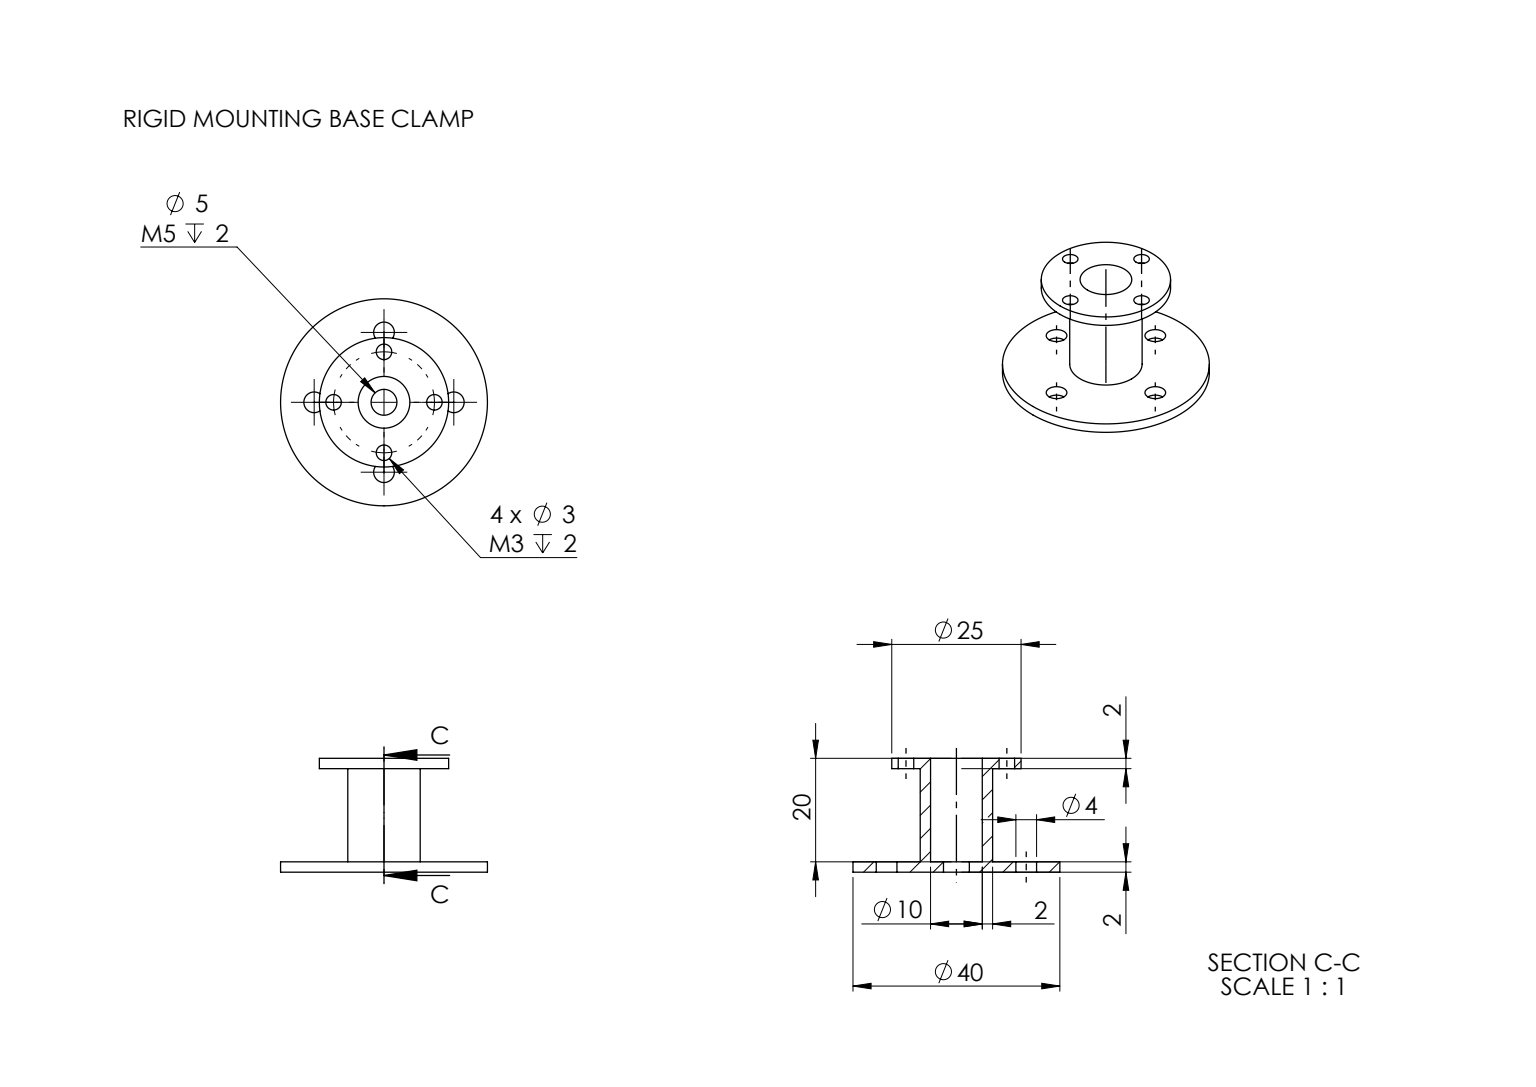
ISO-10303-21;
HEADER;
FILE_DESCRIPTION (('STEP AP214'),
    '1' );
FILE_NAME ('Rigid Mounting Base Clamp.step',
    '2026-10-04T10:31:01',
    ( '' ),
    ( '' ),
    'SwSTEP 2.0',
    'SolidWorks 2026',
    '' );
FILE_SCHEMA (( 'AUTOMOTIVE_DESIGN' ));
ENDSEC;

DATA;
#14=DIRECTION ( 'NONE',  ( 0.000000000000000000, -0.000000000000000000, 1.000000000000000000 ) ) ;
#15=DIRECTION ( 'NONE',  ( 0.000000000000000000, 1.000000000000000000, 0.000000000000000000 ) ) ;
#29=CARTESIAN_POINT ( 'NONE',  ( 8.572527594031473190E-16, 19.99999999999999645, 7.000000000000000000 ) ) ;
#45=CARTESIAN_POINT ( 'NONE',  ( 0.000000000000000000, 22.00000000000000000, -5.000000000000000000 ) ) ;
#61=ORIENTED_EDGE ( 'NONE', *, *, #6502, .F. ) ;
#68=EDGE_CURVE ( 'NONE', #7891, #15426, #13595, .T. ) ;
#80=CYLINDRICAL_SURFACE ( 'NONE', #3453, 2.000000000000000000 ) ;
#135=CARTESIAN_POINT ( 'NONE',  ( 0.000000000000000000, 2.000000000000000000, -5.000000000000000000 ) ) ;
#152=CARTESIAN_POINT ( 'NONE',  ( -13.50000000000000000, -0.001000000000000132727, -1.999999999999997113 ) ) ;
#161=ORIENTED_EDGE ( 'NONE', *, *, #15144, .T. ) ;
#168=FACE_BOUND ( 'NONE', #3506, .T. ) ;
#169=DIRECTION ( 'NONE',  ( 0.000000000000000000, 0.000000000000000000, 1.000000000000000000 ) ) ;
#211=AXIS2_PLACEMENT_3D ( 'NONE', #13271, #4928, #12230 ) ;
#214=FACE_OUTER_BOUND ( 'NONE', #10362, .T. ) ;
#234=CARTESIAN_POINT ( 'NONE',  ( 9.750000000000003553, 19.99999999999999645, 1.020968533498575335E-13 ) ) ;
#237=CYLINDRICAL_SURFACE ( 'NONE', #3717, 2.500000000000000000 ) ;
#238=CARTESIAN_POINT ( 'NONE',  ( 13.50000000000000000, 2.000000000000000000, -2.000000000000000444 ) ) ;
#241=ORIENTED_EDGE ( 'NONE', *, *, #4453, .T. ) ;
#244=AXIS2_PLACEMENT_3D ( 'NONE', #12080, #1179, #6133 ) ;
#246=CIRCLE ( 'NONE', #4794, 1.499999999999999556 ) ;
#275=EDGE_CURVE ( 'NONE', #9042, #302, #14114, .T. ) ;
#302=VERTEX_POINT ( 'NONE', #12936 ) ;
#313=DIRECTION ( 'NONE',  ( 0.000000000000000000, 0.000000000000000000, -1.000000000000000000 ) ) ;
#343=AXIS2_PLACEMENT_3D ( 'NONE', #14019, #15537, #15300 ) ;
#391=AXIS2_PLACEMENT_3D ( 'NONE', #8568, #1379, #7592 ) ;
#450=LINE ( 'NONE', #2848, #4783 ) ;
#460=EDGE_CURVE ( 'NONE', #3041, #9290, #14361, .T. ) ;
#491=AXIS2_PLACEMENT_3D ( 'NONE', #7668, #1615, #14760 ) ;
#538=( LENGTH_UNIT ( ) NAMED_UNIT ( * ) SI_UNIT ( .MILLI., .METRE. ) );
#545=DIRECTION ( 'NONE',  ( -0.000000000000000000, 1.000000000000000000, -0.000000000000000000 ) ) ;
#570=ORIENTED_EDGE ( 'NONE', *, *, #4975, .F. ) ;
#579=CIRCLE ( 'NONE', #3127, 2.500000000000000000 ) ;
#603=DIRECTION ( 'NONE',  ( 0.000000000000000000, 1.000000000000000000, 0.000000000000000000 ) ) ;
#612=VECTOR ( 'NONE', #7149, 1000.000000000000000 ) ;
#635=EDGE_CURVE ( 'NONE', #13364, #1681, #12596, .T. ) ;
#644=DIRECTION ( 'NONE',  ( 0.000000000000000000, 0.000000000000000000, 1.000000000000000000 ) ) ;
#645=VERTEX_POINT ( 'NONE', #6427 ) ;
#662=DIRECTION ( 'NONE',  ( -0.000000000000000000, 1.000000000000000000, -0.000000000000000000 ) ) ;
#688=AXIS2_PLACEMENT_3D ( 'NONE', #3084, #7934, #12777 ) ;
#703=VERTEX_POINT ( 'NONE', #13060 ) ;
#711=AXIS2_PLACEMENT_3D ( 'NONE', #4234, #3121, #10361 ) ;
#722=ORIENTED_EDGE ( 'NONE', *, *, #3306, .T. ) ;
#729=ADVANCED_FACE ( 'NONE', ( #11618 ), #5821, .F. ) ;
#732=CARTESIAN_POINT ( 'NONE',  ( -13.50000000000000000, 0.000000000000000000, 2.479909768273400161E-15 ) ) ;
#750=FACE_OUTER_BOUND ( 'NONE', #5902, .T. ) ;
#756=DIRECTION ( 'NONE',  ( 0.000000000000000000, 1.000000000000000000, 0.000000000000000000 ) ) ;
#769=ORIENTED_EDGE ( 'NONE', *, *, #11126, .T. ) ;
#798=DIRECTION ( 'NONE',  ( -0.000000000000000000, 1.000000000000000000, -0.000000000000000000 ) ) ;
#799=DIRECTION ( 'NONE',  ( 0.000000000000000000, 0.000000000000000000, 1.000000000000000000 ) ) ;
#807=( NAMED_UNIT ( * ) PLANE_ANGLE_UNIT ( ) SI_UNIT ( $, .RADIAN. ) );
#824=ORIENTED_EDGE ( 'NONE', *, *, #635, .T. ) ;
#827=DIRECTION ( 'NONE',  ( 0.000000000000000000, -0.000000000000000000, 1.000000000000000000 ) ) ;
#831=CARTESIAN_POINT ( 'NONE',  ( 0.000000000000000000, 19.99999999999999645, 12.50000000000000355 ) ) ;
#838=ADVANCED_FACE ( 'NONE', ( #7404 ), #80, .F. ) ;
#849=AXIS2_PLACEMENT_3D ( 'NONE', #732, #12900, #2001 ) ;
#852=( NAMED_UNIT ( * ) SI_UNIT ( $, .STERADIAN. ) SOLID_ANGLE_UNIT ( ) );
#866=CARTESIAN_POINT ( 'NONE',  ( 0.000000000000000000, 2.000000000000000000, -2.500000000000000000 ) ) ;
#894=EDGE_LOOP ( 'NONE', ( #6085, #14105 ) ) ;
#901=FACE_BOUND ( 'NONE', #10404, .T. ) ;
#907=CARTESIAN_POINT ( 'NONE',  ( 0.000000000000000000, 0.000000000000000000, 0.000000000000000000 ) ) ;
#919=DIRECTION ( 'NONE',  ( 0.000000000000000000, 1.000000000000000000, 0.000000000000000000 ) ) ;
#929=CARTESIAN_POINT ( 'NONE',  ( -9.750000000000003553, 22.00000000000000000, -1.500000000000033751 ) ) ;
#958=ADVANCED_FACE ( 'NONE', ( #14875 ), #237, .F. ) ;
#959=ORIENTED_EDGE ( 'NONE', *, *, #1371, .T. ) ;
#960=ORIENTED_EDGE ( 'NONE', *, *, #11186, .T. ) ;
#966=CARTESIAN_POINT ( 'NONE',  ( 9.750000000000003553, 22.00000000000000000, 1.500000000000101696 ) ) ;
#977=CIRCLE ( 'NONE', #711, 2.000000000000000000 ) ;
#978=ORIENTED_EDGE ( 'NONE', *, *, #14189, .T. ) ;
#984=DIRECTION ( 'NONE',  ( -0.000000000000000000, 1.000000000000000000, -0.000000000000000000 ) ) ;
#1005=CYLINDRICAL_SURFACE ( 'NONE', #3266, 20.00000000000000000 ) ;
#1031=CARTESIAN_POINT ( 'NONE',  ( 9.750000000000003553, 22.00000000000000000, 1.500000000000101696 ) ) ;
#1038=ORIENTED_EDGE ( 'NONE', *, *, #14388, .F. ) ;
#1040=VERTEX_POINT ( 'NONE', #4128 ) ;
#1044=ORIENTED_EDGE ( 'NONE', *, *, #4453, .F. ) ;
#1069=FACE_OUTER_BOUND ( 'NONE', #8290, .T. ) ;
#1102=CARTESIAN_POINT ( 'NONE',  ( 13.50000000000000000, 0.000000000000000000, 1.999999999999998668 ) ) ;
#1115=DIRECTION ( 'NONE',  ( 0.000000000000000000, 0.000000000000000000, 1.000000000000000000 ) ) ;
#1128=CARTESIAN_POINT ( 'NONE',  ( 2.897581130414634077E-17, 22.00000000000000000, 11.25000000000000355 ) ) ;
#1154=ORIENTED_EDGE ( 'NONE', *, *, #15555, .T. ) ;
#1156=CARTESIAN_POINT ( 'NONE',  ( -9.750000000000003553, 22.00000000000000000, 1.499999999999965583 ) ) ;
#1157=DIRECTION ( 'NONE',  ( 0.000000000000000000, 0.000000000000000000, 1.000000000000000000 ) ) ;
#1166=EDGE_CURVE ( 'NONE', #1681, #6851, #4445, .T. ) ;
#1179=DIRECTION ( 'NONE',  ( -0.000000000000000000, -1.000000000000000000, -0.000000000000000000 ) ) ;
#1180=DIRECTION ( 'NONE',  ( -0.000000000000000000, 1.000000000000000000, -0.000000000000000000 ) ) ;
#1193=ADVANCED_BREP_SHAPE_REPRESENTATION ( '', ( #15484, #14201 ), #5333 ) ;
#1200=CARTESIAN_POINT ( 'NONE',  ( 0.000000000000000000, 2.000000000000000000, 0.000000000000000000 ) ) ;
#1218=CIRCLE ( 'NONE', #5792, 1.499999999999999556 ) ;
#1226=DIRECTION ( 'NONE',  ( 0.000000000000000000, 0.000000000000000000, 1.000000000000000000 ) ) ;
#1291=ORIENTED_EDGE ( 'NONE', *, *, #10850, .F. ) ;
#1306=DIRECTION ( 'NONE',  ( -0.000000000000000000, 1.000000000000000000, -0.000000000000000000 ) ) ;
#1350=ORIENTED_EDGE ( 'NONE', *, *, #8234, .T. ) ;
#1371=EDGE_CURVE ( 'NONE', #4873, #14187, #2186, .T. ) ;
#1379=DIRECTION ( 'NONE',  ( -0.000000000000000000, -1.000000000000000000, -0.000000000000000000 ) ) ;
#1408=ORIENTED_EDGE ( 'NONE', *, *, #10506, .F. ) ;
#1416=DIRECTION ( 'NONE',  ( 0.000000000000000000, 0.000000000000000000, 1.000000000000000000 ) ) ;
#1433=FACE_BOUND ( 'NONE', #12661, .T. ) ;
#1437=DIRECTION ( 'NONE',  ( -0.000000000000000000, 1.000000000000000000, -0.000000000000000000 ) ) ;
#1447=VERTEX_POINT ( 'NONE', #7771 ) ;
#1467=LINE ( 'NONE', #8729, #1486 ) ;
#1486=VECTOR ( 'NONE', #1702, 1000.000000000000000 ) ;
#1495=AXIS2_PLACEMENT_3D ( 'NONE', #5345, #8255, #14967 ) ;
#1509=ORIENTED_EDGE ( 'NONE', *, *, #68, .T. ) ;
#1516=FACE_OUTER_BOUND ( 'NONE', #4435, .T. ) ;
#1528=EDGE_CURVE ( 'NONE', #13930, #12389, #6542, .T. ) ;
#1536=CYLINDRICAL_SURFACE ( 'NONE', #14676, 2.000000000000000000 ) ;
#1548=EDGE_LOOP ( 'NONE', ( #959, #8690, #8357, #5866 ) ) ;
#1551=DIRECTION ( 'NONE',  ( 0.000000000000000000, 0.000000000000000000, 1.000000000000000000 ) ) ;
#1601=DIRECTION ( 'NONE',  ( 0.000000000000000000, 0.000000000000000000, 1.000000000000000000 ) ) ;
#1604=ORIENTED_EDGE ( 'NONE', *, *, #4264, .T. ) ;
#1608=CARTESIAN_POINT ( 'NONE',  ( -2.897581130414634077E-17, 19.99999999999999645, -8.250000000000003553 ) ) ;
#1610=EDGE_CURVE ( 'NONE', #4214, #15156, #15345, .T. ) ;
#1615=DIRECTION ( 'NONE',  ( -0.000000000000000000, 1.000000000000000000, -0.000000000000000000 ) ) ;
#1626=AXIS2_PLACEMENT_3D ( 'NONE', #3473, #1885, #6759 ) ;
#1647=PLANE ( 'NONE',  #4070 ) ;
#1651=DIRECTION ( 'NONE',  ( 1.000000000000000000, 0.000000000000000000, 0.000000000000000000 ) ) ;
#1654=EDGE_CURVE ( 'NONE', #2649, #5182, #11988, .T. ) ;
#1681=VERTEX_POINT ( 'NONE', #3394 ) ;
#1702=DIRECTION ( 'NONE',  ( -0.000000000000000000, -1.000000000000000000, -0.000000000000000000 ) ) ;
#1717=EDGE_CURVE ( 'NONE', #15426, #9324, #13100, .T. ) ;
#1758=ORIENTED_EDGE ( 'NONE', *, *, #2692, .T. ) ;
#1802=EDGE_CURVE ( 'NONE', #2728, #7333, #13264, .T. ) ;
#1806=( NAMED_UNIT ( * ) SI_UNIT ( $, .STERADIAN. ) SOLID_ANGLE_UNIT ( ) );
#1824=AXIS2_PLACEMENT_3D ( 'NONE', #5870, #7799, #10718 ) ;
#1836=ORIENTED_EDGE ( 'NONE', *, *, #6502, .T. ) ;
#1839=DIRECTION ( 'NONE',  ( -0.000000000000000000, -1.000000000000000000, -0.000000000000000000 ) ) ;
#1840=EDGE_LOOP ( 'NONE', ( #5126, #1408 ) ) ;
#1841=DIRECTION ( 'NONE',  ( -0.000000000000000000, 1.000000000000000000, -0.000000000000000000 ) ) ;
#1856=ORIENTED_EDGE ( 'NONE', *, *, #9485, .T. ) ;
#1862=PLANE ( 'NONE',  #13441 ) ;
#1868=CIRCLE ( 'NONE', #9765, 1.499999999999999556 ) ;
#1878=ORIENTED_EDGE ( 'NONE', *, *, #2692, .F. ) ;
#1884=PRESENTATION_STYLE_ASSIGNMENT (( #12780 ) ) ;
#1885=DIRECTION ( 'NONE',  ( -0.000000000000000000, 1.000000000000000000, -0.000000000000000000 ) ) ;
#1937=DIRECTION ( 'NONE',  ( 0.000000000000000000, 0.000000000000000000, 1.000000000000000000 ) ) ;
#1952=DIRECTION ( 'NONE',  ( 0.000000000000000000, 0.000000000000000000, 1.000000000000000000 ) ) ;
#1960=CIRCLE ( 'NONE', #5291, 1.499999999999999556 ) ;
#1983=VECTOR ( 'NONE', #1839, 1000.000000000000000 ) ;
#1986=CARTESIAN_POINT ( 'NONE',  ( 9.750000000000003553, 22.00000000000000000, 1.020968533498575335E-13 ) ) ;
#1991=ORIENTED_EDGE ( 'NONE', *, *, #14241, .F. ) ;
#1996=ORIENTED_EDGE ( 'NONE', *, *, #1610, .T. ) ;
#1999=EDGE_CURVE ( 'NONE', #7891, #6928, #9713, .T. ) ;
#2001=DIRECTION ( 'NONE',  ( 0.000000000000000000, 0.000000000000000000, 1.000000000000000000 ) ) ;
#2017=CYLINDRICAL_SURFACE ( 'NONE', #8633, 7.000000000000000000 ) ;
#2037=CARTESIAN_POINT ( 'NONE',  ( 2.897581130414634077E-17, 19.99999999999999645, 9.750000000000003553 ) ) ;
#2083=VECTOR ( 'NONE', #3978, 1000.000000000000000 ) ;
#2093=FACE_OUTER_BOUND ( 'NONE', #8454, .T. ) ;
#2166=ORIENTED_EDGE ( 'NONE', *, *, #7266, .T. ) ;
#2172=FACE_OUTER_BOUND ( 'NONE', #5920, .T. ) ;
#2184=ORIENTED_EDGE ( 'NONE', *, *, #5963, .T. ) ;
#2186=CIRCLE ( 'NONE', #9077, 12.50000000000000355 ) ;
#2189=ORIENTED_EDGE ( 'NONE', *, *, #14283, .T. ) ;
#2199=DIRECTION ( 'NONE',  ( -0.000000000000000000, 1.000000000000000000, -0.000000000000000000 ) ) ;
#2234=DIRECTION ( 'NONE',  ( -0.000000000000000000, 1.000000000000000000, -0.000000000000000000 ) ) ;
#2255=DIRECTION ( 'NONE',  ( 0.000000000000000000, 0.000000000000000000, -1.000000000000000000 ) ) ;
#2266=ORIENTED_EDGE ( 'NONE', *, *, #1610, .F. ) ;
#2286=ORIENTED_EDGE ( 'NONE', *, *, #7412, .T. ) ;
#2292=EDGE_CURVE ( 'NONE', #7333, #703, #8327, .T. ) ;
#2336=FACE_BOUND ( 'NONE', #14082, .T. ) ;
#2392=ORIENTED_EDGE ( 'NONE', *, *, #11914, .F. ) ;
#2408=ADVANCED_FACE ( 'NONE', ( #8566 ), #1536, .F. ) ;
#2419=FACE_BOUND ( 'NONE', #9726, .T. ) ;
#2481=DIRECTION ( 'NONE',  ( 0.000000000000000000, 0.000000000000000000, 1.000000000000000000 ) ) ;
#2492=VERTEX_POINT ( 'NONE', #7977 ) ;
#2499=CARTESIAN_POINT ( 'NONE',  ( 0.000000000000000000, -0.001000000000000132727, -13.50000000000000000 ) ) ;
#2520=CARTESIAN_POINT ( 'NONE',  ( 0.000000000000000000, 2.000000000000000000, 0.000000000000000000 ) ) ;
#2524=DIRECTION ( 'NONE',  ( 0.000000000000000000, 0.000000000000000000, 1.000000000000000000 ) ) ;
#2528=VECTOR ( 'NONE', #10347, 1000.000000000000000 ) ;
#2554=ORIENTED_EDGE ( 'NONE', *, *, #1166, .F. ) ;
#2559=CARTESIAN_POINT ( 'NONE',  ( 9.750000000000003553, 22.00000000000000000, 1.020968533498575335E-13 ) ) ;
#2569=ORIENTED_EDGE ( 'NONE', *, *, #15274, .T. ) ;
#2570=ORIENTED_EDGE ( 'NONE', *, *, #10476, .T. ) ;
#2572=DIRECTION ( 'NONE',  ( -0.000000000000000000, 1.000000000000000000, -0.000000000000000000 ) ) ;
#2592=DIRECTION ( 'NONE',  ( 0.000000000000000000, 0.000000000000000000, -1.000000000000000000 ) ) ;
#2649=VERTEX_POINT ( 'NONE', #6309 ) ;
#2659=DIRECTION ( 'NONE',  ( -0.000000000000000000, 1.000000000000000000, -0.000000000000000000 ) ) ;
#2678=CIRCLE ( 'NONE', #4715, 2.500000000000000000 ) ;
#2688=AXIS2_PLACEMENT_3D ( 'NONE', #8502, #3466, #1157 ) ;
#2692=EDGE_CURVE ( 'NONE', #6081, #8841, #1960, .T. ) ;
#2702=ADVANCED_FACE ( 'NONE', ( #168, #5029, #1433, #8544, #3589, #11147 ), #8463, .T. ) ;
#2710=ORIENTED_EDGE ( 'NONE', *, *, #6872, .F. ) ;
#2728=VERTEX_POINT ( 'NONE', #13297 ) ;
#2758=DIRECTION ( 'NONE',  ( -0.000000000000000000, 1.000000000000000000, -0.000000000000000000 ) ) ;
#2812=CARTESIAN_POINT ( 'NONE',  ( 0.000000000000000000, 2.000000000000000000, 0.000000000000000000 ) ) ;
#2814=FACE_OUTER_BOUND ( 'NONE', #11179, .T. ) ;
#2832=DIRECTION ( 'NONE',  ( 0.000000000000000000, 0.000000000000000000, 1.000000000000000000 ) ) ;
#2848=CARTESIAN_POINT ( 'NONE',  ( 0.000000000000000000, -0.001000000000000132727, -11.50000000000000000 ) ) ;
#2863=ORIENTED_EDGE ( 'NONE', *, *, #7405, .T. ) ;
#2911=CARTESIAN_POINT ( 'NONE',  ( 0.000000000000000000, 0.000000000000000000, -2.500000000000000000 ) ) ;
#2934=SURFACE_STYLE_FILL_AREA ( #15029 ) ;
#2943=VERTEX_POINT ( 'NONE', #866 ) ;
#2968=DIRECTION ( 'NONE',  ( 0.000000000000000000, 0.000000000000000000, 1.000000000000000000 ) ) ;
#2980=ORIENTED_EDGE ( 'NONE', *, *, #5079, .F. ) ;
#2987=CARTESIAN_POINT ( 'NONE',  ( 0.000000000000000000, 0.000000000000000000, 0.000000000000000000 ) ) ;
#3027=AXIS2_PLACEMENT_3D ( 'NONE', #14925, #4016, #6506 ) ;
#3040=ORIENTED_EDGE ( 'NONE', *, *, #15555, .F. ) ;
#3041=VERTEX_POINT ( 'NONE', #3649 ) ;
#3060=ORIENTED_EDGE ( 'NONE', *, *, #8685, .T. ) ;
#3075=CARTESIAN_POINT ( 'NONE',  ( 0.000000000000000000, 19.99999999999999645, 0.000000000000000000 ) ) ;
#3083=CARTESIAN_POINT ( 'NONE',  ( 2.126728311762493157E-16, 22.00000000000000000, 8.250000000000003553 ) ) ;
#3084=CARTESIAN_POINT ( 'NONE',  ( -9.750000000000003553, 22.00000000000000000, -3.401296724241641415E-14 ) ) ;
#3116=ORIENTED_EDGE ( 'NONE', *, *, #5417, .T. ) ;
#3121=DIRECTION ( 'NONE',  ( 0.000000000000000000, 1.000000000000000000, 0.000000000000000000 ) ) ;
#3127=AXIS2_PLACEMENT_3D ( 'NONE', #13077, #14347, #15560 ) ;
#3139=ORIENTED_EDGE ( 'NONE', *, *, #9122, .T. ) ;
#3144=DIRECTION ( 'NONE',  ( 0.000000000000000000, 1.000000000000000000, 0.000000000000000000 ) ) ;
#3177=DIRECTION ( 'NONE',  ( -0.000000000000000000, 1.000000000000000000, -0.000000000000000000 ) ) ;
#3187=AXIS2_PLACEMENT_3D ( 'NONE', #6012, #3374, #8241 ) ;
#3191=ORIENTED_EDGE ( 'NONE', *, *, #14382, .F. ) ;
#3198=DIRECTION ( 'NONE',  ( -0.000000000000000000, 1.000000000000000000, -0.000000000000000000 ) ) ;
#3201=FACE_OUTER_BOUND ( 'NONE', #9464, .T. ) ;
#3243=DIRECTION ( 'NONE',  ( -0.000000000000000000, 1.000000000000000000, -0.000000000000000000 ) ) ;
#3266=AXIS2_PLACEMENT_3D ( 'NONE', #2520, #13173, #2592 ) ;
#3269=CIRCLE ( 'NONE', #12168, 5.000000000000000000 ) ;
#3306=EDGE_CURVE ( 'NONE', #10357, #11937, #5804, .T. ) ;
#3336=CARTESIAN_POINT ( 'NONE',  ( 2.897581130414634077E-17, 22.00000000000000000, 11.25000000000000355 ) ) ;
#3343=ORIENTED_EDGE ( 'NONE', *, *, #15674, .T. ) ;
#3361=EDGE_LOOP ( 'NONE', ( #8618, #4170 ) ) ;
#3374=DIRECTION ( 'NONE',  ( -0.000000000000000000, 1.000000000000000000, -0.000000000000000000 ) ) ;
#3376=CARTESIAN_POINT ( 'NONE',  ( 2.449293598294708880E-16, 2.000000000000000000, -15.50000000000000000 ) ) ;
#3381=AXIS2_PLACEMENT_3D ( 'NONE', #6549, #12656, #5275 ) ;
#3384=CARTESIAN_POINT ( 'NONE',  ( 0.000000000000000000, 2.000000000000000000, 0.000000000000000000 ) ) ;
#3394=CARTESIAN_POINT ( 'NONE',  ( 1.979652835806277785E-15, 0.000000000000000000, 11.50000000000000000 ) ) ;
#3406=EDGE_CURVE ( 'NONE', #3525, #2649, #14424, .T. ) ;
#3427=DIRECTION ( 'NONE',  ( 0.000000000000000000, 0.000000000000000000, 1.000000000000000000 ) ) ;
#3448=UNCERTAINTY_MEASURE_WITH_UNIT (LENGTH_MEASURE( 1.000000000000000082E-05 ), #15296, 'distance_accuracy_value', 'NONE');
#3453=AXIS2_PLACEMENT_3D ( 'NONE', #12247, #3579, #1115 ) ;
#3466=DIRECTION ( 'NONE',  ( 0.000000000000000000, 1.000000000000000000, 0.000000000000000000 ) ) ;
#3473=CARTESIAN_POINT ( 'NONE',  ( -2.897581130414634077E-17, 22.00000000000000000, -9.750000000000003553 ) ) ;
#3502=AXIS2_PLACEMENT_3D ( 'NONE', #12204, #14265, #1226 ) ;
#3506=EDGE_LOOP ( 'NONE', ( #12428, #1878 ) ) ;
#3525=VERTEX_POINT ( 'NONE', #14154 ) ;
#3549=VERTEX_POINT ( 'NONE', #3336 ) ;
#3579=DIRECTION ( 'NONE',  ( -0.000000000000000000, 1.000000000000000000, -0.000000000000000000 ) ) ;
#3589=FACE_BOUND ( 'NONE', #14008, .T. ) ;
#3592=ADVANCED_FACE ( 'NONE', ( #15441 ), #4619, .F. ) ;
#3594=DIRECTION ( 'NONE',  ( -0.000000000000000000, 1.000000000000000000, -0.000000000000000000 ) ) ;
#3600=VECTOR ( 'NONE', #13706, 1000.000000000000000 ) ;
#3604=VERTEX_POINT ( 'NONE', #15363 ) ;
#3610=DIRECTION ( 'NONE',  ( 0.000000000000000000, 1.000000000000000000, 0.000000000000000000 ) ) ;
#3612=AXIS2_PLACEMENT_3D ( 'NONE', #1200, #15, #4877 ) ;
#3622=CIRCLE ( 'NONE', #14551, 20.00000000000000000 ) ;
#3646=FACE_OUTER_BOUND ( 'NONE', #5498, .T. ) ;
#3649=CARTESIAN_POINT ( 'NONE',  ( 13.50000000000000000, 2.000000000000000000, 1.999999999999998668 ) ) ;
#3678=DIRECTION ( 'NONE',  ( 0.000000000000000000, 0.000000000000000000, -1.000000000000000000 ) ) ;
#3683=CARTESIAN_POINT ( 'NONE',  ( 8.572527594031473190E-16, 2.000000000000000000, 7.000000000000000000 ) ) ;
#3697=CARTESIAN_POINT ( 'NONE',  ( 2.897581130414634077E-17, 19.99999999999999645, 9.750000000000003553 ) ) ;
#3709=CYLINDRICAL_SURFACE ( 'NONE', #12504, 1.499999999999999556 ) ;
#3717=AXIS2_PLACEMENT_3D ( 'NONE', #7635, #6458, #313 ) ;
#3759=ORIENTED_EDGE ( 'NONE', *, *, #10476, .F. ) ;
#3765=EDGE_CURVE ( 'NONE', #15426, #7891, #1218, .T. ) ;
#3779=AXIS2_PLACEMENT_3D ( 'NONE', #12757, #6659, #11490 ) ;
#3787=CARTESIAN_POINT ( 'NONE',  ( 0.000000000000000000, 0.000000000000000000, -2.500000000000000000 ) ) ;
#3793=AXIS2_PLACEMENT_3D ( 'NONE', #14383, #9233, #14067 ) ;
#3810=DIRECTION ( 'NONE',  ( 0.000000000000000000, 1.000000000000000000, 0.000000000000000000 ) ) ;
#3826=CARTESIAN_POINT ( 'NONE',  ( 2.449293598294706513E-15, 2.000000000000000000, 20.00000000000000000 ) ) ;
#3836=ORIENTED_EDGE ( 'NONE', *, *, #13705, .F. ) ;
#3884=DIRECTION ( 'NONE',  ( 0.000000000000000000, 0.000000000000000000, 1.000000000000000000 ) ) ;
#3894=EDGE_CURVE ( 'NONE', #1040, #12333, #4010, .T. ) ;
#3927=AXIS2_PLACEMENT_3D ( 'NONE', #9474, #5977, #5663 ) ;
#3978=DIRECTION ( 'NONE',  ( -0.000000000000000000, -1.000000000000000000, -0.000000000000000000 ) ) ;
#3986=ORIENTED_EDGE ( 'NONE', *, *, #14352, .T. ) ;
#3991=DIRECTION ( 'NONE',  ( 0.000000000000000000, 0.000000000000000000, 1.000000000000000000 ) ) ;
#3992=CARTESIAN_POINT ( 'NONE',  ( 1.530808498934191916E-15, 19.99999999999999645, -12.50000000000000355 ) ) ;
#3993=ORIENTED_EDGE ( 'NONE', *, *, #10195, .F. ) ;
#3998=VECTOR ( 'NONE', #1180, 1000.000000000000000 ) ;
#4004=DIRECTION ( 'NONE',  ( -0.000000000000000000, -1.000000000000000000, -0.000000000000000000 ) ) ;
#4010=CIRCLE ( 'NONE', #12896, 1.499999999999999556 ) ;
#4016=DIRECTION ( 'NONE',  ( 0.000000000000000000, 1.000000000000000000, 0.000000000000000000 ) ) ;
#4018=CIRCLE ( 'NONE', #13431, 1.499999999999999556 ) ;
#4023=DIRECTION ( 'NONE',  ( 0.000000000000000000, 1.000000000000000000, 0.000000000000000000 ) ) ;
#4052=EDGE_LOOP ( 'NONE', ( #13500, #14141, #9232, #10092 ) ) ;
#4070=AXIS2_PLACEMENT_3D ( 'NONE', #15575, #6754, #4357 ) ;
#4123=AXIS2_PLACEMENT_3D ( 'NONE', #12259, #8464, #169 ) ;
#4128=CARTESIAN_POINT ( 'NONE',  ( 9.750000000000003553, 19.99999999999999645, -1.499999999999897415 ) ) ;
#4155=DIRECTION ( 'NONE',  ( -0.000000000000000000, 1.000000000000000000, -0.000000000000000000 ) ) ;
#4170=ORIENTED_EDGE ( 'NONE', *, *, #12599, .T. ) ;
#4175=CIRCLE ( 'NONE', #14322, 1.499999999999999556 ) ;
#4198=EDGE_LOOP ( 'NONE', ( #14714, #12249 ) ) ;
#4214=VERTEX_POINT ( 'NONE', #11863 ) ;
#4234=CARTESIAN_POINT ( 'NONE',  ( 0.000000000000000000, 2.000000000000000000, -13.50000000000000000 ) ) ;
#4235=ORIENTED_EDGE ( 'NONE', *, *, #5424, .F. ) ;
#4258=FACE_BOUND ( 'NONE', #12870, .T. ) ;
#4259=CYLINDRICAL_SURFACE ( 'NONE', #4888, 12.50000000000000355 ) ;
#4264=EDGE_CURVE ( 'NONE', #8559, #13449, #9369, .T. ) ;
#4297=AXIS2_PLACEMENT_3D ( 'NONE', #15276, #3177, #11917 ) ;
#4298=CARTESIAN_POINT ( 'NONE',  ( 9.750000000000003553, 22.00000000000000000, -1.499999999999897415 ) ) ;
#4339=CARTESIAN_POINT ( 'NONE',  ( 0.000000000000000000, 19.99999999999999645, 0.000000000000000000 ) ) ;
#4357=DIRECTION ( 'NONE',  ( 0.000000000000000000, -0.000000000000000000, 1.000000000000000000 ) ) ;
#4361=CARTESIAN_POINT ( 'NONE',  ( 0.000000000000000000, 0.000000000000000000, 0.000000000000000000 ) ) ;
#4372=PRODUCT_DEFINITION_SHAPE ( 'NONE', 'NONE',  #15315 ) ;
#4397=DIRECTION ( 'NONE',  ( 0.000000000000000000, 0.000000000000000000, 1.000000000000000000 ) ) ;
#4402=DIRECTION ( 'NONE',  ( -0.000000000000000000, 1.000000000000000000, -0.000000000000000000 ) ) ;
#4435=EDGE_LOOP ( 'NONE', ( #1044, #6479, #2189, #978 ) ) ;
#4445=LINE ( 'NONE', #14139, #11092 ) ;
#4453=EDGE_CURVE ( 'NONE', #14180, #14110, #1467, .T. ) ;
#4486=ORIENTED_EDGE ( 'NONE', *, *, #1717, .T. ) ;
#4505=VECTOR ( 'NONE', #10333, 1000.000000000000000 ) ;
#4516=SHAPE_REPRESENTATION_RELATIONSHIP ( 'NONE' , 'NONE' ,  #13925, #1193 ) ;
#4541=DIRECTION ( 'NONE',  ( -0.000000000000000000, 1.000000000000000000, -0.000000000000000000 ) ) ;
#4545=CARTESIAN_POINT ( 'NONE',  ( -2.897581130414634077E-17, 22.00000000000000000, -9.750000000000003553 ) ) ;
#4546=ADVANCED_FACE ( 'NONE', ( #14923 ), #13724, .F. ) ;
#4563=COLOUR_RGB ( '', 0.08235294, 0.09019608, 0.10196078) ;
#4570=ORIENTED_EDGE ( 'NONE', *, *, #15674, .F. ) ;
#4575=DIRECTION ( 'NONE',  ( -0.000000000000000000, -1.000000000000000000, -0.000000000000000000 ) ) ;
#4579=CARTESIAN_POINT ( 'NONE',  ( 0.000000000000000000, 19.99999999999999645, 0.000000000000000000 ) ) ;
#4619=CYLINDRICAL_SURFACE ( 'NONE', #13150, 1.499999999999999556 ) ;
#4640=AXIS2_PLACEMENT_3D ( 'NONE', #11069, #13371, #2481 ) ;
#4646=ORIENTED_EDGE ( 'NONE', *, *, #11914, .T. ) ;
#4660=CARTESIAN_POINT ( 'NONE',  ( 1.734723475976807094E-15, -0.001000000000000132727, 15.50000000000000000 ) ) ;
#4675=EDGE_LOOP ( 'NONE', ( #15609, #4772, #7024, #14824 ) ) ;
#4715=AXIS2_PLACEMENT_3D ( 'NONE', #907, #11880, #15400 ) ;
#4720=EDGE_CURVE ( 'NONE', #5689, #2728, #246, .T. ) ;
#4726=ORIENTED_EDGE ( 'NONE', *, *, #14352, .F. ) ;
#4748=ORIENTED_EDGE ( 'NONE', *, *, #15144, .F. ) ;
#4768=PRODUCT ( 'Rigid Mounting Base Clamp', 'Rigid Mounting Base Clamp', '', ( #12823 ) ) ;
#4772=ORIENTED_EDGE ( 'NONE', *, *, #1999, .T. ) ;
#4783=VECTOR ( 'NONE', #8905, 1000.000000000000000 ) ;
#4788=EDGE_LOOP ( 'NONE', ( #3986, #1996, #10651, #6065 ) ) ;
#4794=AXIS2_PLACEMENT_3D ( 'NONE', #10307, #662, #1937 ) ;
#4798=CYLINDRICAL_SURFACE ( 'NONE', #4123, 12.50000000000000355 ) ;
#4801=CARTESIAN_POINT ( 'NONE',  ( 0.000000000000000000, 2.000000000000000000, 0.000000000000000000 ) ) ;
#4811=ORIENTED_EDGE ( 'NONE', *, *, #8453, .T. ) ;
#4817=DIRECTION ( 'NONE',  ( 0.000000000000000000, 0.000000000000000000, 1.000000000000000000 ) ) ;
#4829=DIRECTION ( 'NONE',  ( -0.000000000000000000, 1.000000000000000000, -0.000000000000000000 ) ) ;
#4844=CARTESIAN_POINT ( 'NONE',  ( 0.000000000000000000, 2.000000000000000000, -20.00000000000000000 ) ) ;
#4873=VERTEX_POINT ( 'NONE', #13312 ) ;
#4876=CARTESIAN_POINT ( 'NONE',  ( 0.000000000000000000, 22.00000000000000000, 0.000000000000000000 ) ) ;
#4877=DIRECTION ( 'NONE',  ( 0.000000000000000000, 0.000000000000000000, 1.000000000000000000 ) ) ;
#4888=AXIS2_PLACEMENT_3D ( 'NONE', #4339, #3144, #7996 ) ;
#4896=CARTESIAN_POINT ( 'NONE',  ( 0.000000000000000000, 0.000000000000000000, 0.000000000000000000 ) ) ;
#4898=DIRECTION ( 'NONE',  ( -0.000000000000000000, 1.000000000000000000, -0.000000000000000000 ) ) ;
#4909=AXIS2_PLACEMENT_3D ( 'NONE', #5114, #1437, #13375 ) ;
#4928=DIRECTION ( 'NONE',  ( -0.000000000000000000, 1.000000000000000000, -0.000000000000000000 ) ) ;
#4953=ORIENTED_EDGE ( 'NONE', *, *, #9926, .T. ) ;
#4975=EDGE_CURVE ( 'NONE', #4214, #12581, #3269, .T. ) ;
#4985=DIRECTION ( 'NONE',  ( 0.000000000000000000, 0.000000000000000000, 1.000000000000000000 ) ) ;
#5009=CYLINDRICAL_SURFACE ( 'NONE', #244, 5.000000000000000000 ) ;
#5010=CARTESIAN_POINT ( 'NONE',  ( 1.547212085679566465E-16, 22.00000000000000000, -11.25000000000000355 ) ) ;
#5016=LINE ( 'NONE', #152, #9044 ) ;
#5029=FACE_BOUND ( 'NONE', #7879, .T. ) ;
#5051=CARTESIAN_POINT ( 'NONE',  ( 1.734723475976807094E-15, -0.001000000000000132727, 13.50000000000000000 ) ) ;
#5056=CIRCLE ( 'NONE', #6070, 7.000000000000000000 ) ;
#5075=LINE ( 'NONE', #3787, #612 ) ;
#5079=EDGE_CURVE ( 'NONE', #9324, #6928, #14723, .T. ) ;
#5111=CYLINDRICAL_SURFACE ( 'NONE', #13257, 2.500000000000000000 ) ;
#5114=CARTESIAN_POINT ( 'NONE',  ( -13.50000000000000000, -0.001000000000000132727, 2.479909768273400161E-15 ) ) ;
#5120=ORIENTED_EDGE ( 'NONE', *, *, #14369, .F. ) ;
#5126=ORIENTED_EDGE ( 'NONE', *, *, #5848, .F. ) ;
#5143=ADVANCED_FACE ( 'NONE', ( #7080 ), #15594, .F. ) ;
#5146=CARTESIAN_POINT ( 'NONE',  ( 6.123233995736766282E-16, 2.000000000000000000, 5.000000000000000000 ) ) ;
#5179=ORIENTED_EDGE ( 'NONE', *, *, #15541, .F. ) ;
#5182=VERTEX_POINT ( 'NONE', #10895 ) ;
#5188=LINE ( 'NONE', #3826, #2083 ) ;
#5199=ORIENTED_EDGE ( 'NONE', *, *, #9485, .F. ) ;
#5223=ADVANCED_FACE ( 'NONE', ( #3646 ), #5009, .F. ) ;
#5275=DIRECTION ( 'NONE',  ( 0.000000000000000000, 0.000000000000000000, -1.000000000000000000 ) ) ;
#5286=DIRECTION ( 'NONE',  ( -0.000000000000000000, 1.000000000000000000, -0.000000000000000000 ) ) ;
#5291=AXIS2_PLACEMENT_3D ( 'NONE', #2559, #6232, #14492 ) ;
#5303=AXIS2_PLACEMENT_3D ( 'NONE', #6703, #11614, #15049 ) ;
#5322=CIRCLE ( 'NONE', #13186, 1.499999999999999556 ) ;
#5333=( GEOMETRIC_REPRESENTATION_CONTEXT ( 3 ) GLOBAL_UNCERTAINTY_ASSIGNED_CONTEXT ( ( #13155 ) ) GLOBAL_UNIT_ASSIGNED_CONTEXT ( ( #538, #13981, #1806 ) ) REPRESENTATION_CONTEXT ( 'NONE', 'WORKASPACE' ) );
#5339=CARTESIAN_POINT ( 'NONE',  ( 0.000000000000000000, 19.99999999999999645, 0.000000000000000000 ) ) ;
#5345=CARTESIAN_POINT ( 'NONE',  ( 0.000000000000000000, 2.000000000000000000, 0.000000000000000000 ) ) ;
#5360=ORIENTED_EDGE ( 'NONE', *, *, #460, .T. ) ;
#5367=SURFACE_STYLE_USAGE ( .BOTH. , #10443 ) ;
#5368=LINE ( 'NONE', #12354, #3600 ) ;
#5377=ADVANCED_FACE ( 'NONE', ( #13658, #7865, #12705, #12550, #15026, #13818 ), #1647, .F. ) ;
#5398=AXIS2_PLACEMENT_3D ( 'NONE', #4896, #13314, #2255 ) ;
#5406=DIRECTION ( 'NONE',  ( 0.000000000000000000, 0.000000000000000000, 1.000000000000000000 ) ) ;
#5407=VECTOR ( 'NONE', #13403, 1000.000000000000000 ) ;
#5417=EDGE_CURVE ( 'NONE', #12389, #13930, #12955, .T. ) ;
#5424=EDGE_CURVE ( 'NONE', #12389, #3604, #15337, .T. ) ;
#5439=DIRECTION ( 'NONE',  ( 0.000000000000000000, 1.000000000000000000, 0.000000000000000000 ) ) ;
#5441=EDGE_LOOP ( 'NONE', ( #9445, #6963, #3343, #10496 ) ) ;
#5442=DIRECTION ( 'NONE',  ( 0.000000000000000000, 0.000000000000000000, 1.000000000000000000 ) ) ;
#5471=CARTESIAN_POINT ( 'NONE',  ( 1.734723475976807094E-15, 2.000000000000000000, 13.50000000000000000 ) ) ;
#5498=EDGE_LOOP ( 'NONE', ( #2266, #6543, #11700, #12194 ) ) ;
#5510=CARTESIAN_POINT ( 'NONE',  ( -13.50000000000000000, 2.000000000000000000, -1.999999999999997113 ) ) ;
#5521=CYLINDRICAL_SURFACE ( 'NONE', #7469, 1.499999999999999556 ) ;
#5546=CIRCLE ( 'NONE', #211, 1.499999999999999556 ) ;
#5556=CIRCLE ( 'NONE', #15202, 1.999999999999999556 ) ;
#5582=LINE ( 'NONE', #9906, #2528 ) ;
#5615=DIRECTION ( 'NONE',  ( 0.000000000000000000, 1.000000000000000000, 0.000000000000000000 ) ) ;
#5635=VERTEX_POINT ( 'NONE', #6029 ) ;
#5663=DIRECTION ( 'NONE',  ( 0.000000000000000000, 0.000000000000000000, 1.000000000000000000 ) ) ;
#5669=ORIENTED_EDGE ( 'NONE', *, *, #3765, .F. ) ;
#5672=VERTEX_POINT ( 'NONE', #2911 ) ;
#5678=AXIS2_PLACEMENT_3D ( 'NONE', #4545, #8047, #799 ) ;
#5689=VERTEX_POINT ( 'NONE', #7761 ) ;
#5700=CARTESIAN_POINT ( 'NONE',  ( 0.000000000000000000, 2.000000000000000000, 0.000000000000000000 ) ) ;
#5759=ADVANCED_FACE ( 'NONE', ( #2172 ), #4259, .T. ) ;
#5770=FACE_BOUND ( 'NONE', #6870, .T. ) ;
#5771=ORIENTED_EDGE ( 'NONE', *, *, #6124, .F. ) ;
#5792=AXIS2_PLACEMENT_3D ( 'NONE', #9947, #12169, #10903 ) ;
#5796=DIRECTION ( 'NONE',  ( -0.000000000000000000, 1.000000000000000000, -0.000000000000000000 ) ) ;
#5804=CIRCLE ( 'NONE', #3502, 12.50000000000000355 ) ;
#5821=CYLINDRICAL_SURFACE ( 'NONE', #14125, 1.999999999999999556 ) ;
#5848=EDGE_CURVE ( 'NONE', #5672, #13817, #12746, .T. ) ;
#5866=ORIENTED_EDGE ( 'NONE', *, *, #6453, .F. ) ;
#5869=ORIENTED_EDGE ( 'NONE', *, *, #7266, .F. ) ;
#5870=CARTESIAN_POINT ( 'NONE',  ( 0.000000000000000000, 22.00000000000000000, 0.000000000000000000 ) ) ;
#5874=FACE_OUTER_BOUND ( 'NONE', #11847, .T. ) ;
#5894=DIRECTION ( 'NONE',  ( 0.000000000000000000, 0.000000000000000000, 1.000000000000000000 ) ) ;
#5902=EDGE_LOOP ( 'NONE', ( #3993, #4570 ) ) ;
#5920=EDGE_LOOP ( 'NONE', ( #14750, #1856, #9838, #5771 ) ) ;
#5943=CARTESIAN_POINT ( 'NONE',  ( 9.750000000000003553, 22.00000000000000000, 1.020968533498575335E-13 ) ) ;
#5963=EDGE_CURVE ( 'NONE', #13449, #3041, #5368, .T. ) ;
#5968=CIRCLE ( 'NONE', #11538, 2.000000000000000000 ) ;
#5977=DIRECTION ( 'NONE',  ( -0.000000000000000000, -1.000000000000000000, -0.000000000000000000 ) ) ;
#5989=CARTESIAN_POINT ( 'NONE',  ( -9.750000000000003553, 22.00000000000000000, -1.500000000000033751 ) ) ;
#5998=ORIENTED_EDGE ( 'NONE', *, *, #1371, .F. ) ;
#6012=CARTESIAN_POINT ( 'NONE',  ( 0.000000000000000000, -0.001000000000000132727, -13.50000000000000000 ) ) ;
#6013=AXIS2_PLACEMENT_3D ( 'NONE', #12451, #8969, #1551 ) ;
#6024=CARTESIAN_POINT ( 'NONE',  ( 3.061616997868383141E-16, 0.000000000000000000, 2.500000000000000000 ) ) ;
#6029=CARTESIAN_POINT ( 'NONE',  ( 2.449293598294708880E-16, 0.000000000000000000, -15.50000000000000000 ) ) ;
#6065=ORIENTED_EDGE ( 'NONE', *, *, #13730, .F. ) ;
#6069=ORIENTED_EDGE ( 'NONE', *, *, #10113, .F. ) ;
#6070=AXIS2_PLACEMENT_3D ( 'NONE', #3384, #7296, #9685 ) ;
#6076=CYLINDRICAL_SURFACE ( 'NONE', #4909, 1.999999999999999556 ) ;
#6080=CARTESIAN_POINT ( 'NONE',  ( 9.750000000000003553, 19.99999999999999645, 1.500000000000101696 ) ) ;
#6081=VERTEX_POINT ( 'NONE', #4298 ) ;
#6085=ORIENTED_EDGE ( 'NONE', *, *, #635, .F. ) ;
#6108=AXIS2_PLACEMENT_3D ( 'NONE', #7601, #13487, #2832 ) ;
#6117=CARTESIAN_POINT ( 'NONE',  ( 9.750000000000003553, 22.00000000000000000, 1.020968533498575335E-13 ) ) ;
#6121=VECTOR ( 'NONE', #9447, 1000.000000000000000 ) ;
#6124=EDGE_CURVE ( 'NONE', #11937, #10357, #9718, .T. ) ;
#6133=DIRECTION ( 'NONE',  ( 0.000000000000000000, 0.000000000000000000, -1.000000000000000000 ) ) ;
#6165=CIRCLE ( 'NONE', #9960, 7.000000000000000000 ) ;
#6170=LINE ( 'NONE', #7661, #10378 ) ;
#6225=ORIENTED_EDGE ( 'NONE', *, *, #275, .F. ) ;
#6230=ORIENTED_EDGE ( 'NONE', *, *, #1802, .F. ) ;
#6232=DIRECTION ( 'NONE',  ( -0.000000000000000000, 1.000000000000000000, -0.000000000000000000 ) ) ;
#6252=PLANE ( 'NONE',  #10221 ) ;
#6300=PRODUCT_DEFINITION_FORMATION_WITH_SPECIFIED_SOURCE ( 'ANY', '', #4768, .NOT_KNOWN. ) ;
#6309=CARTESIAN_POINT ( 'NONE',  ( 0.000000000000000000, 2.000000000000000000, -20.00000000000000000 ) ) ;
#6312=DIRECTION ( 'NONE',  ( 0.000000000000000000, 0.000000000000000000, -1.000000000000000000 ) ) ;
#6336=VECTOR ( 'NONE', #14442, 1000.000000000000000 ) ;
#6379=CARTESIAN_POINT ( 'NONE',  ( 0.000000000000000000, 2.000000000000000000, -7.000000000000000000 ) ) ;
#6414=LINE ( 'NONE', #10428, #12176 ) ;
#6427=CARTESIAN_POINT ( 'NONE',  ( -13.50000000000000000, 0.000000000000000000, -1.999999999999997113 ) ) ;
#6436=DIRECTION ( 'NONE',  ( 0.000000000000000000, 0.000000000000000000, 1.000000000000000000 ) ) ;
#6446=VERTEX_POINT ( 'NONE', #8159 ) ;
#6449=CIRCLE ( 'NONE', #5678, 1.499999999999999556 ) ;
#6453=EDGE_CURVE ( 'NONE', #4873, #10357, #11727, .T. ) ;
#6458=DIRECTION ( 'NONE',  ( -0.000000000000000000, -1.000000000000000000, -0.000000000000000000 ) ) ;
#6467=DIRECTION ( 'NONE',  ( 0.000000000000000000, 1.000000000000000000, 0.000000000000000000 ) ) ;
#6468=EDGE_LOOP ( 'NONE', ( #11219, #3116 ) ) ;
#6479=ORIENTED_EDGE ( 'NONE', *, *, #9122, .F. ) ;
#6481=ORIENTED_EDGE ( 'NONE', *, *, #7412, .F. ) ;
#6493=CARTESIAN_POINT ( 'NONE',  ( 0.000000000000000000, 0.000000000000000000, -13.50000000000000000 ) ) ;
#6502=EDGE_CURVE ( 'NONE', #14180, #6446, #6165, .T. ) ;
#6506=DIRECTION ( 'NONE',  ( 0.000000000000000000, 0.000000000000000000, 1.000000000000000000 ) ) ;
#6542=CIRCLE ( 'NONE', #15422, 1.499999999999999556 ) ;
#6543=ORIENTED_EDGE ( 'NONE', *, *, #4975, .T. ) ;
#6549=CARTESIAN_POINT ( 'NONE',  ( 0.000000000000000000, 2.000000000000000000, 0.000000000000000000 ) ) ;
#6558=ORIENTED_EDGE ( 'NONE', *, *, #9926, .F. ) ;
#6560=ADVANCED_FACE ( 'NONE', ( #2336, #2419, #12201, #8318, #13157, #9755 ), #6252, .T. ) ;
#6632=AXIS2_PLACEMENT_3D ( 'NONE', #2037, #11670, #10484 ) ;
#6633=CARTESIAN_POINT ( 'NONE',  ( 0.000000000000000000, 19.99999999999999645, 0.000000000000000000 ) ) ;
#6659=DIRECTION ( 'NONE',  ( -0.000000000000000000, -1.000000000000000000, -0.000000000000000000 ) ) ;
#6680=CARTESIAN_POINT ( 'NONE',  ( 0.000000000000000000, 0.000000000000000000, 0.000000000000000000 ) ) ;
#6686=LINE ( 'NONE', #7710, #11021 ) ;
#6703=CARTESIAN_POINT ( 'NONE',  ( 0.000000000000000000, 2.000000000000000000, 0.000000000000000000 ) ) ;
#6715=FILL_AREA_STYLE ('',( #15141 ) ) ;
#6729=ADVANCED_FACE ( 'NONE', ( #9887 ), #5111, .F. ) ;
#6736=ADVANCED_FACE ( 'NONE', ( #1516 ), #11305, .T. ) ;
#6754=DIRECTION ( 'NONE',  ( 0.000000000000000000, 1.000000000000000000, 0.000000000000000000 ) ) ;
#6759=DIRECTION ( 'NONE',  ( 0.000000000000000000, 0.000000000000000000, 1.000000000000000000 ) ) ;
#6767=ORIENTED_EDGE ( 'NONE', *, *, #1528, .F. ) ;
#6777=CARTESIAN_POINT ( 'NONE',  ( 1.547212085679566958E-16, 22.00000000000000000, -11.25000000000000355 ) ) ;
#6801=SHAPE_DEFINITION_REPRESENTATION ( #4372, #13925 ) ;
#6843=CIRCLE ( 'NONE', #7096, 2.000000000000000000 ) ;
#6851=VERTEX_POINT ( 'NONE', #12338 ) ;
#6853=( GEOMETRIC_REPRESENTATION_CONTEXT ( 3 ) GLOBAL_UNCERTAINTY_ASSIGNED_CONTEXT ( ( #8565 ) ) GLOBAL_UNIT_ASSIGNED_CONTEXT ( ( #15417, #11985, #852 ) ) REPRESENTATION_CONTEXT ( 'NONE', 'WORKASPACE' ) );
#6870=EDGE_LOOP ( 'NONE', ( #6069, #6481 ) ) ;
#6872=EDGE_CURVE ( 'NONE', #3525, #10771, #5188, .T. ) ;
#6897=DIRECTION ( 'NONE',  ( 0.000000000000000000, 0.000000000000000000, 1.000000000000000000 ) ) ;
#6928=VERTEX_POINT ( 'NONE', #6777 ) ;
#6963=ORIENTED_EDGE ( 'NONE', *, *, #6872, .T. ) ;
#6980=EDGE_CURVE ( 'NONE', #10964, #13817, #15203, .T. ) ;
#6999=EDGE_LOOP ( 'NONE', ( #14469, #10592, #9420, #8536 ) ) ;
#7024=ORIENTED_EDGE ( 'NONE', *, *, #9248, .T. ) ;
#7045=DIRECTION ( 'NONE',  ( 0.000000000000000000, 1.000000000000000000, 0.000000000000000000 ) ) ;
#7046=DIRECTION ( 'NONE',  ( -0.000000000000000000, 1.000000000000000000, -0.000000000000000000 ) ) ;
#7048=CARTESIAN_POINT ( 'NONE',  ( 1.547212085679566958E-16, 19.99999999999999645, -11.25000000000000355 ) ) ;
#7080=FACE_OUTER_BOUND ( 'NONE', #11718, .T. ) ;
#7096=AXIS2_PLACEMENT_3D ( 'NONE', #9920, #10156, #8970 ) ;
#7149=DIRECTION ( 'NONE',  ( -0.000000000000000000, -1.000000000000000000, -0.000000000000000000 ) ) ;
#7174=CARTESIAN_POINT ( 'NONE',  ( -2.897581130414634077E-17, 22.00000000000000000, -8.250000000000003553 ) ) ;
#7179=EDGE_LOOP ( 'NONE', ( #8305, #9306 ) ) ;
#7191=VECTOR ( 'NONE', #3594, 1000.000000000000000 ) ;
#7196=ORIENTED_EDGE ( 'NONE', *, *, #7936, .F. ) ;
#7203=AXIS2_PLACEMENT_3D ( 'NONE', #6633, #11464, #1601 ) ;
#7255=ORIENTED_EDGE ( 'NONE', *, *, #8453, .F. ) ;
#7258=ORIENTED_EDGE ( 'NONE', *, *, #10506, .T. ) ;
#7266=EDGE_CURVE ( 'NONE', #5689, #703, #10869, .T. ) ;
#7273=CARTESIAN_POINT ( 'NONE',  ( 0.000000000000000000, 22.00000000000000000, 0.000000000000000000 ) ) ;
#7296=DIRECTION ( 'NONE',  ( 0.000000000000000000, 1.000000000000000000, 0.000000000000000000 ) ) ;
#7313=ADVANCED_FACE ( 'NONE', ( #12024 ), #4798, .T. ) ;
#7333=VERTEX_POINT ( 'NONE', #5989 ) ;
#7337=CIRCLE ( 'NONE', #11893, 7.000000000000000000 ) ;
#7343=FACE_OUTER_BOUND ( 'NONE', #13230, .T. ) ;
#7349=ORIENTED_EDGE ( 'NONE', *, *, #6124, .T. ) ;
#7356=DIRECTION ( 'NONE',  ( 0.000000000000000000, 0.000000000000000000, 1.000000000000000000 ) ) ;
#7404=FACE_OUTER_BOUND ( 'NONE', #9010, .T. ) ;
#7405=EDGE_CURVE ( 'NONE', #15156, #12174, #10478, .T. ) ;
#7412=EDGE_CURVE ( 'NONE', #645, #9501, #11491, .T. ) ;
#7443=AXIS2_PLACEMENT_3D ( 'NONE', #4801, #9890, #14661 ) ;
#7452=FACE_OUTER_BOUND ( 'NONE', #4675, .T. ) ;
#7462=ADVANCED_FACE ( 'NONE', ( #7569 ), #11673, .F. ) ;
#7469=AXIS2_PLACEMENT_3D ( 'NONE', #15219, #4402, #3427 ) ;
#7495=CARTESIAN_POINT ( 'NONE',  ( 13.50000000000000000, 0.000000000000000000, -2.000000000000000444 ) ) ;
#7521=EDGE_LOOP ( 'NONE', ( #7196, #10589, #7258, #15684 ) ) ;
#7569=FACE_OUTER_BOUND ( 'NONE', #8870, .T. ) ;
#7582=DIRECTION ( 'NONE',  ( 0.000000000000000000, 1.000000000000000000, 0.000000000000000000 ) ) ;
#7592=DIRECTION ( 'NONE',  ( 0.000000000000000000, 0.000000000000000000, -1.000000000000000000 ) ) ;
#7599=EDGE_LOOP ( 'NONE', ( #13365, #3836 ) ) ;
#7601=CARTESIAN_POINT ( 'NONE',  ( 2.897581130414634077E-17, 22.00000000000000000, 9.750000000000003553 ) ) ;
#7626=ADVANCED_FACE ( 'NONE', ( #214 ), #8814, .F. ) ;
#7635=CARTESIAN_POINT ( 'NONE',  ( 0.000000000000000000, 0.000000000000000000, 0.000000000000000000 ) ) ;
#7637=ORIENTED_EDGE ( 'NONE', *, *, #15480, .T. ) ;
#7661=CARTESIAN_POINT ( 'NONE',  ( 13.50000000000000000, -0.001000000000000132727, -2.000000000000000444 ) ) ;
#7668=CARTESIAN_POINT ( 'NONE',  ( 2.897581130414634077E-17, 22.00000000000000000, 9.750000000000003553 ) ) ;
#7688=CARTESIAN_POINT ( 'NONE',  ( -9.750000000000003553, 22.00000000000000000, -3.401296724241641415E-14 ) ) ;
#7693=ADVANCED_FACE ( 'NONE', ( #7452 ), #3709, .F. ) ;
#7710=CARTESIAN_POINT ( 'NONE',  ( 1.530808498934191916E-15, 19.99999999999999645, -12.50000000000000355 ) ) ;
#7714=EDGE_LOOP ( 'NONE', ( #5179, #14687, #8949, #11294 ) ) ;
#7761=CARTESIAN_POINT ( 'NONE',  ( -9.750000000000003553, 19.99999999999999645, 1.499999999999965583 ) ) ;
#7771=CARTESIAN_POINT ( 'NONE',  ( 0.000000000000000000, 0.000000000000000000, -11.50000000000000000 ) ) ;
#7799=DIRECTION ( 'NONE',  ( 0.000000000000000000, 1.000000000000000000, 0.000000000000000000 ) ) ;
#7817=AXIS2_PLACEMENT_3D ( 'NONE', #4361, #10098, #5406 ) ;
#7858=STYLED_ITEM ( 'NONE', ( #8055 ), #15484 ) ;
#7865=FACE_BOUND ( 'NONE', #9749, .T. ) ;
#7879=EDGE_LOOP ( 'NONE', ( #2980, #9916 ) ) ;
#7884=EDGE_CURVE ( 'NONE', #2649, #3525, #3622, .T. ) ;
#7891=VERTEX_POINT ( 'NONE', #7048 ) ;
#7914=DIRECTION ( 'NONE',  ( 0.000000000000000000, 0.000000000000000000, -1.000000000000000000 ) ) ;
#7934=DIRECTION ( 'NONE',  ( -0.000000000000000000, 1.000000000000000000, -0.000000000000000000 ) ) ;
#7936=EDGE_CURVE ( 'NONE', #10964, #2943, #579, .T. ) ;
#7939=SURFACE_SIDE_STYLE ('',( #2934 ) ) ;
#7972=DIRECTION ( 'NONE',  ( -0.000000000000000000, -1.000000000000000000, -0.000000000000000000 ) ) ;
#7977=CARTESIAN_POINT ( 'NONE',  ( 1.734723475976807094E-15, 2.000000000000000000, 15.50000000000000000 ) ) ;
#7996=DIRECTION ( 'NONE',  ( 0.000000000000000000, 0.000000000000000000, 1.000000000000000000 ) ) ;
#8014=VERTEX_POINT ( 'NONE', #3376 ) ;
#8028=EDGE_LOOP ( 'NONE', ( #824, #12429, #161, #3759 ) ) ;
#8047=DIRECTION ( 'NONE',  ( -0.000000000000000000, 1.000000000000000000, -0.000000000000000000 ) ) ;
#8055=PRESENTATION_STYLE_ASSIGNMENT (( #5367 ) ) ;
#8068=EDGE_LOOP ( 'NONE', ( #4235, #6767, #4811, #7637 ) ) ;
#8159=CARTESIAN_POINT ( 'NONE',  ( 0.000000000000000000, 19.99999999999999645, -7.000000000000000000 ) ) ;
#8192=ORIENTED_EDGE ( 'NONE', *, *, #5424, .T. ) ;
#8232=CIRCLE ( 'NONE', #849, 1.999999999999999556 ) ;
#8234=EDGE_CURVE ( 'NONE', #5635, #1447, #15069, .T. ) ;
#8241=DIRECTION ( 'NONE',  ( 0.000000000000000000, 0.000000000000000000, 1.000000000000000000 ) ) ;
#8255=DIRECTION ( 'NONE',  ( 0.000000000000000000, 1.000000000000000000, 0.000000000000000000 ) ) ;
#8290=EDGE_LOOP ( 'NONE', ( #1038, #1350, #11139, #14035 ) ) ;
#8305=ORIENTED_EDGE ( 'NONE', *, *, #15480, .F. ) ;
#8318=FACE_BOUND ( 'NONE', #11684, .T. ) ;
#8327=CIRCLE ( 'NONE', #688, 1.499999999999999556 ) ;
#8345=CARTESIAN_POINT ( 'NONE',  ( -2.897581130414634077E-17, 22.00000000000000000, -8.250000000000003553 ) ) ;
#8357=ORIENTED_EDGE ( 'NONE', *, *, #3306, .F. ) ;
#8453=EDGE_CURVE ( 'NONE', #13930, #3549, #10835, .T. ) ;
#8454=EDGE_LOOP ( 'NONE', ( #61, #241, #8480, #9898 ) ) ;
#8463=PLANE ( 'NONE',  #10111 ) ;
#8464=DIRECTION ( 'NONE',  ( 0.000000000000000000, 1.000000000000000000, 0.000000000000000000 ) ) ;
#8474=DIRECTION ( 'NONE',  ( -0.000000000000000000, -1.000000000000000000, -0.000000000000000000 ) ) ;
#8476=FACE_OUTER_BOUND ( 'NONE', #4788, .T. ) ;
#8480=ORIENTED_EDGE ( 'NONE', *, *, #13705, .T. ) ;
#8491=ADVANCED_FACE ( 'NONE', ( #7343 ), #6076, .F. ) ;
#8502=CARTESIAN_POINT ( 'NONE',  ( 13.50000000000000000, 2.000000000000000000, -8.673617379884035472E-16 ) ) ;
#8536=ORIENTED_EDGE ( 'NONE', *, *, #5963, .F. ) ;
#8544=FACE_BOUND ( 'NONE', #7179, .T. ) ;
#8545=AXIS2_PLACEMENT_3D ( 'NONE', #14722, #3810, #1416 ) ;
#8550=EDGE_CURVE ( 'NONE', #12174, #15156, #12266, .T. ) ;
#8559=VERTEX_POINT ( 'NONE', #7495 ) ;
#8563=FACE_OUTER_BOUND ( 'NONE', #11587, .T. ) ;
#8565=UNCERTAINTY_MEASURE_WITH_UNIT (LENGTH_MEASURE( 1.000000000000000082E-05 ), #15417, 'distance_accuracy_value', 'NONE');
#8566=FACE_OUTER_BOUND ( 'NONE', #8028, .T. ) ;
#8568=CARTESIAN_POINT ( 'NONE',  ( 0.000000000000000000, 2.000000000000000000, 0.000000000000000000 ) ) ;
#8586=CARTESIAN_POINT ( 'NONE',  ( -2.897581130414634077E-17, 22.00000000000000000, -9.750000000000003553 ) ) ;
#8590=VECTOR ( 'NONE', #13022, 1000.000000000000000 ) ;
#8614=EDGE_LOOP ( 'NONE', ( #722, #7349 ) ) ;
#8618=ORIENTED_EDGE ( 'NONE', *, *, #4720, .T. ) ;
#8633=AXIS2_PLACEMENT_3D ( 'NONE', #15160, #4575, #7914 ) ;
#8644=CIRCLE ( 'NONE', #491, 1.499999999999999556 ) ;
#8685=EDGE_CURVE ( 'NONE', #2943, #10964, #13032, .T. ) ;
#8690=ORIENTED_EDGE ( 'NONE', *, *, #9440, .T. ) ;
#8699=CARTESIAN_POINT ( 'NONE',  ( 0.000000000000000000, 22.00000000000000000, 0.000000000000000000 ) ) ;
#8712=DIRECTION ( 'NONE',  ( 1.000000000000000000, 0.000000000000000000, 0.000000000000000000 ) ) ;
#8729=CARTESIAN_POINT ( 'NONE',  ( 8.572527594031473190E-16, 22.00000000000000000, 7.000000000000000000 ) ) ;
#8737=DIRECTION ( 'NONE',  ( -0.000000000000000000, 1.000000000000000000, -0.000000000000000000 ) ) ;
#8814=CYLINDRICAL_SURFACE ( 'NONE', #13776, 1.499999999999999556 ) ;
#8831=VECTOR ( 'NONE', #5796, 1000.000000000000000 ) ;
#8841=VERTEX_POINT ( 'NONE', #1031 ) ;
#8847=ORIENTED_EDGE ( 'NONE', *, *, #8550, .T. ) ;
#8870=EDGE_LOOP ( 'NONE', ( #11701, #13255, #15338, #3040 ) ) ;
#8872=AXIS2_PLACEMENT_3D ( 'NONE', #10684, #8474, #9494 ) ;
#8905=DIRECTION ( 'NONE',  ( -0.000000000000000000, 1.000000000000000000, -0.000000000000000000 ) ) ;
#8949=ORIENTED_EDGE ( 'NONE', *, *, #10190, .T. ) ;
#8969=DIRECTION ( 'NONE',  ( -0.000000000000000000, -1.000000000000000000, -0.000000000000000000 ) ) ;
#8970=DIRECTION ( 'NONE',  ( 0.000000000000000000, 0.000000000000000000, 1.000000000000000000 ) ) ;
#9004=AXIS2_PLACEMENT_3D ( 'NONE', #5339, #10260, #9081 ) ;
#9010=EDGE_LOOP ( 'NONE', ( #2554, #2569, #2570, #769 ) ) ;
#9027=CARTESIAN_POINT ( 'NONE',  ( 13.50000000000000000, 0.000000000000000000, -8.673617379884035472E-16 ) ) ;
#9035=CARTESIAN_POINT ( 'NONE',  ( 2.449293598294706513E-15, 0.000000000000000000, 20.00000000000000000 ) ) ;
#9042=VERTEX_POINT ( 'NONE', #5510 ) ;
#9044=VECTOR ( 'NONE', #12397, 1000.000000000000000 ) ;
#9053=AXIS2_PLACEMENT_3D ( 'NONE', #11814, #919, #14126 ) ;
#9077=AXIS2_PLACEMENT_3D ( 'NONE', #3075, #603, #12697 ) ;
#9081=DIRECTION ( 'NONE',  ( 0.000000000000000000, 0.000000000000000000, 1.000000000000000000 ) ) ;
#9102=LINE ( 'NONE', #12813, #15725 ) ;
#9122=EDGE_CURVE ( 'NONE', #6446, #14180, #12026, .T. ) ;
#9160=FACE_OUTER_BOUND ( 'NONE', #15114, .T. ) ;
#9232=ORIENTED_EDGE ( 'NONE', *, *, #11062, .T. ) ;
#9233=DIRECTION ( 'NONE',  ( -0.000000000000000000, 1.000000000000000000, -0.000000000000000000 ) ) ;
#9238=CARTESIAN_POINT ( 'NONE',  ( 3.061616997868383141E-16, 0.000000000000000000, 2.500000000000000000 ) ) ;
#9244=AXIS2_PLACEMENT_3D ( 'NONE', #9360, #14199, #1952 ) ;
#9248=EDGE_CURVE ( 'NONE', #6928, #9324, #6449, .T. ) ;
#9290=VERTEX_POINT ( 'NONE', #238 ) ;
#9306=ORIENTED_EDGE ( 'NONE', *, *, #15588, .F. ) ;
#9324=VERTEX_POINT ( 'NONE', #7174 ) ;
#9347=ORIENTED_EDGE ( 'NONE', *, *, #4264, .F. ) ;
#9360=CARTESIAN_POINT ( 'NONE',  ( -13.50000000000000000, 2.000000000000000000, 2.479909768273400161E-15 ) ) ;
#9369=CIRCLE ( 'NONE', #8872, 1.999999999999999556 ) ;
#9383=EDGE_LOOP ( 'NONE', ( #9895, #11649 ) ) ;
#9389=DIRECTION ( 'NONE',  ( -0.000000000000000000, -1.000000000000000000, -0.000000000000000000 ) ) ;
#9420=ORIENTED_EDGE ( 'NONE', *, *, #15100, .T. ) ;
#9426=EDGE_CURVE ( 'NONE', #12333, #1040, #1868, .T. ) ;
#9430=DIRECTION ( 'NONE',  ( 0.000000000000000000, 0.000000000000000000, 1.000000000000000000 ) ) ;
#9440=EDGE_CURVE ( 'NONE', #14187, #11937, #6686, .T. ) ;
#9445=ORIENTED_EDGE ( 'NONE', *, *, #3406, .F. ) ;
#9447=DIRECTION ( 'NONE',  ( -0.000000000000000000, 1.000000000000000000, -0.000000000000000000 ) ) ;
#9464=EDGE_LOOP ( 'NONE', ( #12270, #8192, #15549, #7255 ) ) ;
#9474=CARTESIAN_POINT ( 'NONE',  ( 0.000000000000000000, 0.000000000000000000, -13.50000000000000000 ) ) ;
#9475=CARTESIAN_POINT ( 'NONE',  ( 13.50000000000000000, -0.001000000000000132727, -8.673617379884035472E-16 ) ) ;
#9479=ORIENTED_EDGE ( 'NONE', *, *, #2292, .T. ) ;
#9485=EDGE_CURVE ( 'NONE', #14187, #4873, #14574, .T. ) ;
#9494=DIRECTION ( 'NONE',  ( 0.000000000000000000, 0.000000000000000000, 1.000000000000000000 ) ) ;
#9498=VERTEX_POINT ( 'NONE', #6379 ) ;
#9501=VERTEX_POINT ( 'NONE', #13829 ) ;
#9524=ORIENTED_EDGE ( 'NONE', *, *, #14388, .T. ) ;
#9525=CYLINDRICAL_SURFACE ( 'NONE', #13134, 1.999999999999999556 ) ;
#9543=VECTOR ( 'NONE', #7046, 1000.000000000000000 ) ;
#9685=DIRECTION ( 'NONE',  ( 1.000000000000000000, 0.000000000000000000, 0.000000000000000000 ) ) ;
#9713=LINE ( 'NONE', #5010, #3998 ) ;
#9718=CIRCLE ( 'NONE', #1824, 12.50000000000000355 ) ;
#9726=EDGE_LOOP ( 'NONE', ( #9937, #13506 ) ) ;
#9749=EDGE_LOOP ( 'NONE', ( #12598, #1509 ) ) ;
#9755=FACE_OUTER_BOUND ( 'NONE', #9383, .T. ) ;
#9757=FACE_OUTER_BOUND ( 'NONE', #10569, .T. ) ;
#9765=AXIS2_PLACEMENT_3D ( 'NONE', #11444, #545, #13754 ) ;
#9771=DIRECTION ( 'NONE',  ( -0.000000000000000000, 1.000000000000000000, -0.000000000000000000 ) ) ;
#9803=ORIENTED_EDGE ( 'NONE', *, *, #10190, .F. ) ;
#9838=ORIENTED_EDGE ( 'NONE', *, *, #6453, .T. ) ;
#9878=EDGE_LOOP ( 'NONE', ( #12432, #4748 ) ) ;
#9887=FACE_OUTER_BOUND ( 'NONE', #7521, .T. ) ;
#9890=DIRECTION ( 'NONE',  ( 0.000000000000000000, 1.000000000000000000, 0.000000000000000000 ) ) ;
#9895=ORIENTED_EDGE ( 'NONE', *, *, #7884, .T. ) ;
#9898=ORIENTED_EDGE ( 'NONE', *, *, #14283, .F. ) ;
#9906=CARTESIAN_POINT ( 'NONE',  ( 9.750000000000003553, 22.00000000000000000, -1.499999999999897415 ) ) ;
#9916=ORIENTED_EDGE ( 'NONE', *, *, #9248, .F. ) ;
#9920=CARTESIAN_POINT ( 'NONE',  ( 1.734723475976807094E-15, 2.000000000000000000, 13.50000000000000000 ) ) ;
#9926=EDGE_CURVE ( 'NONE', #302, #9042, #10018, .T. ) ;
#9937=ORIENTED_EDGE ( 'NONE', *, *, #460, .F. ) ;
#9947=CARTESIAN_POINT ( 'NONE',  ( -2.897581130414634077E-17, 19.99999999999999645, -9.750000000000003553 ) ) ;
#9960=AXIS2_PLACEMENT_3D ( 'NONE', #4579, #7045, #9430 ) ;
#9964=CARTESIAN_POINT ( 'NONE',  ( 0.000000000000000000, 0.000000000000000000, 0.000000000000000000 ) ) ;
#9994=AXIS2_PLACEMENT_3D ( 'NONE', #6493, #4004, #10143 ) ;
#10018=CIRCLE ( 'NONE', #9244, 1.999999999999999556 ) ;
#10092=ORIENTED_EDGE ( 'NONE', *, *, #5848, .T. ) ;
#10098=DIRECTION ( 'NONE',  ( 0.000000000000000000, 1.000000000000000000, 0.000000000000000000 ) ) ;
#10111=AXIS2_PLACEMENT_3D ( 'NONE', #4876, #12181, #14 ) ;
#10113=EDGE_CURVE ( 'NONE', #9501, #645, #8232, .T. ) ;
#10143=DIRECTION ( 'NONE',  ( 0.000000000000000000, 0.000000000000000000, 1.000000000000000000 ) ) ;
#10156=DIRECTION ( 'NONE',  ( 0.000000000000000000, 1.000000000000000000, 0.000000000000000000 ) ) ;
#10187=ADVANCED_FACE ( 'NONE', ( #3201 ), #5521, .F. ) ;
#10190=EDGE_CURVE ( 'NONE', #12333, #8841, #15378, .T. ) ;
#10195=EDGE_CURVE ( 'NONE', #5182, #10771, #14307, .T. ) ;
#10221=AXIS2_PLACEMENT_3D ( 'NONE', #14598, #3610, #13241 ) ;
#10233=VECTOR ( 'NONE', #9389, 1000.000000000000000 ) ;
#10239=DIRECTION ( 'NONE',  ( 0.000000000000000000, 0.000000000000000000, 1.000000000000000000 ) ) ;
#10260=DIRECTION ( 'NONE',  ( 0.000000000000000000, 1.000000000000000000, 0.000000000000000000 ) ) ;
#10264=ORIENTED_EDGE ( 'NONE', *, *, #15541, .T. ) ;
#10307=CARTESIAN_POINT ( 'NONE',  ( -9.750000000000003553, 19.99999999999999645, -3.401296724241641415E-14 ) ) ;
#10333=DIRECTION ( 'NONE',  ( -0.000000000000000000, -1.000000000000000000, -0.000000000000000000 ) ) ;
#10337=DIRECTION ( 'NONE',  ( 0.000000000000000000, 1.000000000000000000, 0.000000000000000000 ) ) ;
#10347=DIRECTION ( 'NONE',  ( -0.000000000000000000, 1.000000000000000000, -0.000000000000000000 ) ) ;
#10357=VERTEX_POINT ( 'NONE', #13438 ) ;
#10361=DIRECTION ( 'NONE',  ( 0.000000000000000000, 0.000000000000000000, 1.000000000000000000 ) ) ;
#10362=EDGE_LOOP ( 'NONE', ( #13346, #10264, #1758, #9803 ) ) ;
#10364=( NAMED_UNIT ( * ) SI_UNIT ( $, .STERADIAN. ) SOLID_ANGLE_UNIT ( ) );
#10378=VECTOR ( 'NONE', #5286, 1000.000000000000000 ) ;
#10404=EDGE_LOOP ( 'NONE', ( #2392, #10828 ) ) ;
#10408=CARTESIAN_POINT ( 'NONE',  ( -13.50000000000000000, -0.001000000000000132727, 2.479909768273400161E-15 ) ) ;
#10428=CARTESIAN_POINT ( 'NONE',  ( -13.50000000000000000, -0.001000000000000132727, 2.000000000000002220 ) ) ;
#10443=SURFACE_SIDE_STYLE ('',( #11706 ) ) ;
#10476=EDGE_CURVE ( 'NONE', #13364, #2492, #14514, .T. ) ;
#10478=CIRCLE ( 'NONE', #3612, 5.000000000000000000 ) ;
#10484=DIRECTION ( 'NONE',  ( 0.000000000000000000, 0.000000000000000000, 1.000000000000000000 ) ) ;
#10496=ORIENTED_EDGE ( 'NONE', *, *, #1654, .F. ) ;
#10506=EDGE_CURVE ( 'NONE', #13817, #5672, #2678, .T. ) ;
#10512=VECTOR ( 'NONE', #2234, 1000.000000000000000 ) ;
#10569=EDGE_LOOP ( 'NONE', ( #2710, #12832, #14398, #11061 ) ) ;
#10575=ADVANCED_FACE ( 'NONE', ( #1069 ), #10779, .F. ) ;
#10589=ORIENTED_EDGE ( 'NONE', *, *, #6980, .T. ) ;
#10592=ORIENTED_EDGE ( 'NONE', *, *, #14241, .T. ) ;
#10635=EDGE_LOOP ( 'NONE', ( #3139, #1836 ) ) ;
#10651=ORIENTED_EDGE ( 'NONE', *, *, #8550, .F. ) ;
#10665=ADVANCED_FACE ( 'NONE', ( #9757 ), #12439, .T. ) ;
#10684=CARTESIAN_POINT ( 'NONE',  ( 13.50000000000000000, 0.000000000000000000, -8.673617379884035472E-16 ) ) ;
#10715=FACE_OUTER_BOUND ( 'NONE', #5441, .T. ) ;
#10718=DIRECTION ( 'NONE',  ( 0.000000000000000000, 0.000000000000000000, 1.000000000000000000 ) ) ;
#10721=CYLINDRICAL_SURFACE ( 'NONE', #1626, 1.499999999999999556 ) ;
#10729=CARTESIAN_POINT ( 'NONE',  ( 0.000000000000000000, 2.000000000000000000, -11.50000000000000000 ) ) ;
#10771=VERTEX_POINT ( 'NONE', #9035 ) ;
#10779=CYLINDRICAL_SURFACE ( 'NONE', #3187, 2.000000000000000000 ) ;
#10788=DIRECTION ( 'NONE',  ( 0.000000000000000000, 0.000000000000000000, 1.000000000000000000 ) ) ;
#10798=CARTESIAN_POINT ( 'NONE',  ( 3.061616997868383141E-16, 2.000000000000000000, 2.500000000000000000 ) ) ;
#10828=ORIENTED_EDGE ( 'NONE', *, *, #8234, .F. ) ;
#10835=LINE ( 'NONE', #1128, #7191 ) ;
#10845=ORIENTED_EDGE ( 'NONE', *, *, #11186, .F. ) ;
#10846=EDGE_CURVE ( 'NONE', #645, #9042, #5016, .T. ) ;
#10850=EDGE_CURVE ( 'NONE', #8014, #12563, #13083, .T. ) ;
#10869=LINE ( 'NONE', #1156, #5407 ) ;
#10872=FACE_OUTER_BOUND ( 'NONE', #13910, .T. ) ;
#10895=CARTESIAN_POINT ( 'NONE',  ( 0.000000000000000000, 0.000000000000000000, -20.00000000000000000 ) ) ;
#10903=DIRECTION ( 'NONE',  ( 0.000000000000000000, 0.000000000000000000, 1.000000000000000000 ) ) ;
#10923=CARTESIAN_POINT ( 'NONE',  ( 2.126728311762493650E-16, 19.99999999999999645, 8.250000000000003553 ) ) ;
#10954=DIRECTION ( 'NONE',  ( 0.000000000000000000, 0.000000000000000000, 1.000000000000000000 ) ) ;
#10959=ADVANCED_FACE ( 'NONE', ( #5874 ), #10721, .F. ) ;
#10964=VERTEX_POINT ( 'NONE', #10798 ) ;
#11003=CYLINDRICAL_SURFACE ( 'NONE', #11550, 5.000000000000000000 ) ;
#11021=VECTOR ( 'NONE', #10337, 1000.000000000000000 ) ;
#11025=LINE ( 'NONE', #45, #6336 ) ;
#11061=ORIENTED_EDGE ( 'NONE', *, *, #10195, .T. ) ;
#11062=EDGE_CURVE ( 'NONE', #2943, #5672, #5075, .T. ) ;
#11069=CARTESIAN_POINT ( 'NONE',  ( -13.50000000000000000, 0.000000000000000000, 2.479909768273400161E-15 ) ) ;
#11070=DIRECTION ( 'NONE',  ( 0.000000000000000000, 0.000000000000000000, -1.000000000000000000 ) ) ;
#11092=VECTOR ( 'NONE', #3243, 1000.000000000000000 ) ;
#11126=EDGE_CURVE ( 'NONE', #2492, #6851, #5968, .T. ) ;
#11139=ORIENTED_EDGE ( 'NONE', *, *, #12695, .T. ) ;
#11147=FACE_OUTER_BOUND ( 'NONE', #8614, .T. ) ;
#11179=EDGE_LOOP ( 'NONE', ( #6230, #11470, #2166, #960 ) ) ;
#11186=EDGE_CURVE ( 'NONE', #703, #7333, #4175, .T. ) ;
#11219=ORIENTED_EDGE ( 'NONE', *, *, #1528, .T. ) ;
#11294=ORIENTED_EDGE ( 'NONE', *, *, #13727, .T. ) ;
#11305=CYLINDRICAL_SURFACE ( 'NONE', #15058, 7.000000000000000000 ) ;
#11374=PLANE ( 'NONE',  #1495 ) ;
#11404=CIRCLE ( 'NONE', #3779, 2.000000000000000000 ) ;
#11444=CARTESIAN_POINT ( 'NONE',  ( 9.750000000000003553, 19.99999999999999645, 1.020968533498575335E-13 ) ) ;
#11464=DIRECTION ( 'NONE',  ( 0.000000000000000000, 1.000000000000000000, 0.000000000000000000 ) ) ;
#11470=ORIENTED_EDGE ( 'NONE', *, *, #4720, .F. ) ;
#11490=DIRECTION ( 'NONE',  ( 0.000000000000000000, 0.000000000000000000, 1.000000000000000000 ) ) ;
#11491=CIRCLE ( 'NONE', #4640, 1.999999999999999556 ) ;
#11500=PRODUCT_DEFINITION_CONTEXT ( 'detailed design', #13184, 'design' ) ;
#11513=DIRECTION ( 'NONE',  ( 0.000000000000000000, 0.000000000000000000, 1.000000000000000000 ) ) ;
#11538=AXIS2_PLACEMENT_3D ( 'NONE', #5471, #4023, #10239 ) ;
#11550=AXIS2_PLACEMENT_3D ( 'NONE', #7273, #15703, #3678 ) ;
#11562=CLOSED_SHELL ( 'NONE', ( #6729, #7626, #7693, #5143, #10187, #12316, #7313, #15388, #729, #2408, #7462, #15056, #15229, #6736, #10665, #6560, #15232, #8491, #838, #15001, #10575, #5759, #5377, #14754, #5223, #2702, #4546, #15467, #10959, #3592, #958 ) ) ;
#11587=EDGE_LOOP ( 'NONE', ( #4646, #9524, #13542, #11915 ) ) ;
#11605=FACE_BOUND ( 'NONE', #11869, .T. ) ;
#11607=VECTOR ( 'NONE', #2199, 1000.000000000000000 ) ;
#11614=DIRECTION ( 'NONE',  ( 0.000000000000000000, 1.000000000000000000, 0.000000000000000000 ) ) ;
#11618=FACE_OUTER_BOUND ( 'NONE', #6999, .T. ) ;
#11649=ORIENTED_EDGE ( 'NONE', *, *, #3406, .T. ) ;
#11651=CIRCLE ( 'NONE', #3027, 1.999999999999999556 ) ;
#11670=DIRECTION ( 'NONE',  ( -0.000000000000000000, 1.000000000000000000, -0.000000000000000000 ) ) ;
#11673=CYLINDRICAL_SURFACE ( 'NONE', #13525, 1.999999999999999556 ) ;
#11684=EDGE_LOOP ( 'NONE', ( #6558, #6225 ) ) ;
#11700=ORIENTED_EDGE ( 'NONE', *, *, #13730, .T. ) ;
#11701=ORIENTED_EDGE ( 'NONE', *, *, #10113, .T. ) ;
#11706=SURFACE_STYLE_FILL_AREA ( #6715 ) ;
#11718=EDGE_LOOP ( 'NONE', ( #13384, #13775, #9479, #5869 ) ) ;
#11727=LINE ( 'NONE', #831, #11979 ) ;
#11814=CARTESIAN_POINT ( 'NONE',  ( -13.50000000000000000, 2.000000000000000000, 2.479909768273400161E-15 ) ) ;
#11847=EDGE_LOOP ( 'NONE', ( #13839, #5669, #4486, #15198 ) ) ;
#11863=CARTESIAN_POINT ( 'NONE',  ( 6.123233995736766282E-16, 22.00000000000000000, 5.000000000000000000 ) ) ;
#11869=EDGE_LOOP ( 'NONE', ( #3060, #11911 ) ) ;
#11880=DIRECTION ( 'NONE',  ( -0.000000000000000000, -1.000000000000000000, -0.000000000000000000 ) ) ;
#11893=AXIS2_PLACEMENT_3D ( 'NONE', #2812, #7582, #8712 ) ;
#11907=MECHANICAL_DESIGN_GEOMETRIC_PRESENTATION_REPRESENTATION('',(#7858),#14444);
#11911=ORIENTED_EDGE ( 'NONE', *, *, #7936, .T. ) ;
#11914=EDGE_CURVE ( 'NONE', #1447, #5635, #12565, .T. ) ;
#11915=ORIENTED_EDGE ( 'NONE', *, *, #12695, .F. ) ;
#11917=DIRECTION ( 'NONE',  ( 0.000000000000000000, 0.000000000000000000, 1.000000000000000000 ) ) ;
#11937=VERTEX_POINT ( 'NONE', #14559 ) ;
#11979=VECTOR ( 'NONE', #12994, 1000.000000000000000 ) ;
#11985=( NAMED_UNIT ( * ) PLANE_ANGLE_UNIT ( ) SI_UNIT ( $, .RADIAN. ) );
#11988=LINE ( 'NONE', #4844, #8590 ) ;
#12021=ORIENTED_EDGE ( 'NONE', *, *, #10846, .F. ) ;
#12024=FACE_OUTER_BOUND ( 'NONE', #1548, .T. ) ;
#12026=CIRCLE ( 'NONE', #7203, 7.000000000000000000 ) ;
#12080=CARTESIAN_POINT ( 'NONE',  ( 0.000000000000000000, 22.00000000000000000, 0.000000000000000000 ) ) ;
#12165=AXIS2_PLACEMENT_3D ( 'NONE', #2499, #984, #7356 ) ;
#12168=AXIS2_PLACEMENT_3D ( 'NONE', #12488, #6467, #13838 ) ;
#12169=DIRECTION ( 'NONE',  ( -0.000000000000000000, 1.000000000000000000, -0.000000000000000000 ) ) ;
#12174=VERTEX_POINT ( 'NONE', #135 ) ;
#12176=VECTOR ( 'NONE', #2659, 1000.000000000000000 ) ;
#12181=DIRECTION ( 'NONE',  ( 0.000000000000000000, 1.000000000000000000, 0.000000000000000000 ) ) ;
#12194=ORIENTED_EDGE ( 'NONE', *, *, #7405, .F. ) ;
#12201=FACE_BOUND ( 'NONE', #9878, .T. ) ;
#12204=CARTESIAN_POINT ( 'NONE',  ( 0.000000000000000000, 22.00000000000000000, 0.000000000000000000 ) ) ;
#12230=DIRECTION ( 'NONE',  ( 0.000000000000000000, 0.000000000000000000, 1.000000000000000000 ) ) ;
#12247=CARTESIAN_POINT ( 'NONE',  ( 1.734723475976807094E-15, -0.001000000000000132727, 13.50000000000000000 ) ) ;
#12249=ORIENTED_EDGE ( 'NONE', *, *, #3894, .T. ) ;
#12259=CARTESIAN_POINT ( 'NONE',  ( 0.000000000000000000, 19.99999999999999645, 0.000000000000000000 ) ) ;
#12260=DIRECTION ( 'NONE',  ( -0.000000000000000000, -1.000000000000000000, -0.000000000000000000 ) ) ;
#12266=CIRCLE ( 'NONE', #7443, 5.000000000000000000 ) ;
#12270=ORIENTED_EDGE ( 'NONE', *, *, #5417, .F. ) ;
#12297=DIRECTION ( 'NONE',  ( -0.000000000000000000, 1.000000000000000000, -0.000000000000000000 ) ) ;
#12316=ADVANCED_FACE ( 'NONE', ( #8476 ), #11003, .F. ) ;
#12333=VERTEX_POINT ( 'NONE', #6080 ) ;
#12338=CARTESIAN_POINT ( 'NONE',  ( 1.979652835806277785E-15, 2.000000000000000000, 11.50000000000000000 ) ) ;
#12354=CARTESIAN_POINT ( 'NONE',  ( 13.50000000000000000, -0.001000000000000132727, 1.999999999999998668 ) ) ;
#12389=VERTEX_POINT ( 'NONE', #10923 ) ;
#12397=DIRECTION ( 'NONE',  ( -0.000000000000000000, 1.000000000000000000, -0.000000000000000000 ) ) ;
#12427=STYLED_ITEM ( 'NONE', ( #1884 ), #1193 ) ;
#12428=ORIENTED_EDGE ( 'NONE', *, *, #13727, .F. ) ;
#12429=ORIENTED_EDGE ( 'NONE', *, *, #1166, .T. ) ;
#12432=ORIENTED_EDGE ( 'NONE', *, *, #11126, .F. ) ;
#12439=CYLINDRICAL_SURFACE ( 'NONE', #391, 20.00000000000000000 ) ;
#12451=CARTESIAN_POINT ( 'NONE',  ( 1.734723475976807094E-15, 0.000000000000000000, 13.50000000000000000 ) ) ;
#12488=CARTESIAN_POINT ( 'NONE',  ( 0.000000000000000000, 22.00000000000000000, 0.000000000000000000 ) ) ;
#12504=AXIS2_PLACEMENT_3D ( 'NONE', #8586, #12297, #2524 ) ;
#12550=FACE_BOUND ( 'NONE', #6468, .T. ) ;
#12563=VERTEX_POINT ( 'NONE', #10729 ) ;
#12565=CIRCLE ( 'NONE', #3927, 2.000000000000000000 ) ;
#12575=AXIS2_PLACEMENT_3D ( 'NONE', #14903, #2572, #3991 ) ;
#12581=VERTEX_POINT ( 'NONE', #14466 ) ;
#12585=CARTESIAN_POINT ( 'NONE',  ( 0.000000000000000000, 22.00000000000000000, -7.000000000000000000 ) ) ;
#12596=CIRCLE ( 'NONE', #6013, 2.000000000000000000 ) ;
#12598=ORIENTED_EDGE ( 'NONE', *, *, #3765, .T. ) ;
#12599=EDGE_CURVE ( 'NONE', #2728, #5689, #5546, .T. ) ;
#12656=DIRECTION ( 'NONE',  ( -0.000000000000000000, -1.000000000000000000, -0.000000000000000000 ) ) ;
#12661=EDGE_LOOP ( 'NONE', ( #10845, #13833 ) ) ;
#12695=EDGE_CURVE ( 'NONE', #1447, #12563, #450, .T. ) ;
#12697=DIRECTION ( 'NONE',  ( 0.000000000000000000, 0.000000000000000000, 1.000000000000000000 ) ) ;
#12705=FACE_BOUND ( 'NONE', #3361, .T. ) ;
#12739=CARTESIAN_POINT ( 'NONE',  ( 2.897581130414634077E-17, 22.00000000000000000, 9.750000000000003553 ) ) ;
#12746=CIRCLE ( 'NONE', #5398, 2.500000000000000000 ) ;
#12757=CARTESIAN_POINT ( 'NONE',  ( 1.734723475976807094E-15, 0.000000000000000000, 13.50000000000000000 ) ) ;
#12777=DIRECTION ( 'NONE',  ( 0.000000000000000000, 0.000000000000000000, 1.000000000000000000 ) ) ;
#12780=SURFACE_STYLE_USAGE ( .BOTH. , #7939 ) ;
#12813=CARTESIAN_POINT ( 'NONE',  ( 2.449293598294707893E-16, -0.001000000000000132727, -15.50000000000000000 ) ) ;
#12815=CARTESIAN_POINT ( 'NONE',  ( -9.750000000000003553, 22.00000000000000000, -3.401296724241641415E-14 ) ) ;
#12823=PRODUCT_CONTEXT ( 'NONE', #13696, 'mechanical' ) ;
#12832=ORIENTED_EDGE ( 'NONE', *, *, #7884, .F. ) ;
#12870=EDGE_LOOP ( 'NONE', ( #3191, #9347 ) ) ;
#12891=CARTESIAN_POINT ( 'NONE',  ( 0.000000000000000000, 22.00000000000000000, 0.000000000000000000 ) ) ;
#12896=AXIS2_PLACEMENT_3D ( 'NONE', #234, #14799, #3884 ) ;
#12900=DIRECTION ( 'NONE',  ( -0.000000000000000000, -1.000000000000000000, -0.000000000000000000 ) ) ;
#12936=CARTESIAN_POINT ( 'NONE',  ( -13.50000000000000000, 2.000000000000000000, 2.000000000000002220 ) ) ;
#12955=CIRCLE ( 'NONE', #6632, 1.499999999999999556 ) ;
#12964=DIRECTION ( 'NONE',  ( 0.000000000000000000, 0.000000000000000000, 1.000000000000000000 ) ) ;
#12994=DIRECTION ( 'NONE',  ( 0.000000000000000000, 1.000000000000000000, 0.000000000000000000 ) ) ;
#13022=DIRECTION ( 'NONE',  ( -0.000000000000000000, -1.000000000000000000, -0.000000000000000000 ) ) ;
#13032=CIRCLE ( 'NONE', #3381, 2.500000000000000000 ) ;
#13060=CARTESIAN_POINT ( 'NONE',  ( -9.750000000000003553, 22.00000000000000000, 1.499999999999965583 ) ) ;
#13077=CARTESIAN_POINT ( 'NONE',  ( 0.000000000000000000, 2.000000000000000000, 0.000000000000000000 ) ) ;
#13083=CIRCLE ( 'NONE', #8545, 2.000000000000000000 ) ;
#13100=LINE ( 'NONE', #8345, #11607 ) ;
#13134=AXIS2_PLACEMENT_3D ( 'NONE', #14691, #9771, #14528 ) ;
#13150=AXIS2_PLACEMENT_3D ( 'NONE', #1986, #4541, #5894 ) ;
#13155=UNCERTAINTY_MEASURE_WITH_UNIT (LENGTH_MEASURE( 1.000000000000000082E-05 ), #538, 'distance_accuracy_value', 'NONE');
#13157=FACE_BOUND ( 'NONE', #7599, .T. ) ;
#13173=DIRECTION ( 'NONE',  ( -0.000000000000000000, -1.000000000000000000, -0.000000000000000000 ) ) ;
#13184=APPLICATION_CONTEXT ( 'automotive_design' ) ;
#13186=AXIS2_PLACEMENT_3D ( 'NONE', #12739, #1841, #2968 ) ;
#13230=EDGE_LOOP ( 'NONE', ( #12021, #2286, #1154, #4953 ) ) ;
#13241=DIRECTION ( 'NONE',  ( 0.000000000000000000, -0.000000000000000000, 1.000000000000000000 ) ) ;
#13255=ORIENTED_EDGE ( 'NONE', *, *, #10846, .T. ) ;
#13257=AXIS2_PLACEMENT_3D ( 'NONE', #9964, #12260, #11070 ) ;
#13264=LINE ( 'NONE', #929, #8831 ) ;
#13271=CARTESIAN_POINT ( 'NONE',  ( -9.750000000000003553, 19.99999999999999645, -3.401296724241641415E-14 ) ) ;
#13297=CARTESIAN_POINT ( 'NONE',  ( -9.750000000000003553, 19.99999999999999645, -1.500000000000033751 ) ) ;
#13312=CARTESIAN_POINT ( 'NONE',  ( 0.000000000000000000, 19.99999999999999645, 12.50000000000000355 ) ) ;
#13314=DIRECTION ( 'NONE',  ( -0.000000000000000000, -1.000000000000000000, -0.000000000000000000 ) ) ;
#13346=ORIENTED_EDGE ( 'NONE', *, *, #3894, .F. ) ;
#13364=VERTEX_POINT ( 'NONE', #15271 ) ;
#13365=ORIENTED_EDGE ( 'NONE', *, *, #14189, .F. ) ;
#13371=DIRECTION ( 'NONE',  ( -0.000000000000000000, -1.000000000000000000, -0.000000000000000000 ) ) ;
#13375=DIRECTION ( 'NONE',  ( 0.000000000000000000, 0.000000000000000000, 1.000000000000000000 ) ) ;
#13384=ORIENTED_EDGE ( 'NONE', *, *, #12599, .F. ) ;
#13389=CYLINDRICAL_SURFACE ( 'NONE', #12165, 2.000000000000000000 ) ;
#13403=DIRECTION ( 'NONE',  ( -0.000000000000000000, 1.000000000000000000, -0.000000000000000000 ) ) ;
#13431=AXIS2_PLACEMENT_3D ( 'NONE', #5943, #4829, #10788 ) ;
#13438=CARTESIAN_POINT ( 'NONE',  ( 0.000000000000000000, 22.00000000000000000, 12.50000000000000355 ) ) ;
#13441=AXIS2_PLACEMENT_3D ( 'NONE', #2987, #5615, #827 ) ;
#13449=VERTEX_POINT ( 'NONE', #1102 ) ;
#13451=MECHANICAL_DESIGN_GEOMETRIC_PRESENTATION_REPRESENTATION('',(#12427),#6853);
#13487=DIRECTION ( 'NONE',  ( -0.000000000000000000, 1.000000000000000000, -0.000000000000000000 ) ) ;
#13500=ORIENTED_EDGE ( 'NONE', *, *, #6980, .F. ) ;
#13506=ORIENTED_EDGE ( 'NONE', *, *, #15100, .F. ) ;
#13525=AXIS2_PLACEMENT_3D ( 'NONE', #10408, #15340, #14971 ) ;
#13542=ORIENTED_EDGE ( 'NONE', *, *, #10850, .T. ) ;
#13560=CARTESIAN_POINT ( 'NONE',  ( 2.897581130414634077E-17, 19.99999999999999645, 11.25000000000000355 ) ) ;
#13595=CIRCLE ( 'NONE', #12575, 1.499999999999999556 ) ;
#13658=FACE_BOUND ( 'NONE', #4198, .T. ) ;
#13696=APPLICATION_CONTEXT ( 'automotive_design' ) ;
#13705=EDGE_CURVE ( 'NONE', #14110, #9498, #5056, .T. ) ;
#13706=DIRECTION ( 'NONE',  ( -0.000000000000000000, 1.000000000000000000, -0.000000000000000000 ) ) ;
#13724=CYLINDRICAL_SURFACE ( 'NONE', #6108, 1.499999999999999556 ) ;
#13727=EDGE_CURVE ( 'NONE', #8841, #6081, #4018, .T. ) ;
#13730=EDGE_CURVE ( 'NONE', #12581, #12174, #11025, .T. ) ;
#13754=DIRECTION ( 'NONE',  ( 0.000000000000000000, 0.000000000000000000, 1.000000000000000000 ) ) ;
#13775=ORIENTED_EDGE ( 'NONE', *, *, #1802, .T. ) ;
#13776=AXIS2_PLACEMENT_3D ( 'NONE', #6117, #2758, #10954 ) ;
#13782=CYLINDRICAL_SURFACE ( 'NONE', #14720, 1.499999999999999556 ) ;
#13817=VERTEX_POINT ( 'NONE', #6024 ) ;
#13818=FACE_OUTER_BOUND ( 'NONE', #14882, .T. ) ;
#13829=CARTESIAN_POINT ( 'NONE',  ( -13.50000000000000000, 0.000000000000000000, 2.000000000000002220 ) ) ;
#13833=ORIENTED_EDGE ( 'NONE', *, *, #2292, .F. ) ;
#13838=DIRECTION ( 'NONE',  ( 0.000000000000000000, 0.000000000000000000, 1.000000000000000000 ) ) ;
#13839=ORIENTED_EDGE ( 'NONE', *, *, #1999, .F. ) ;
#13842=DIRECTION ( 'NONE',  ( -0.000000000000000000, -1.000000000000000000, -0.000000000000000000 ) ) ;
#13852=LINE ( 'NONE', #12585, #1983 ) ;
#13902=CARTESIAN_POINT ( 'NONE',  ( 6.123233995736766282E-16, 22.00000000000000000, 5.000000000000000000 ) ) ;
#13910=EDGE_LOOP ( 'NONE', ( #1991, #1604, #2184, #5360 ) ) ;
#13925=SHAPE_REPRESENTATION ( 'Rigid Mounting Base Clamp', ( #14201 ), #5333 ) ;
#13930=VERTEX_POINT ( 'NONE', #13560 ) ;
#13981=( NAMED_UNIT ( * ) PLANE_ANGLE_UNIT ( ) SI_UNIT ( $, .RADIAN. ) );
#14008=EDGE_LOOP ( 'NONE', ( #4726, #570 ) ) ;
#14019=CARTESIAN_POINT ( 'NONE',  ( 0.000000000000000000, 0.000000000000000000, 0.000000000000000000 ) ) ;
#14033=FACE_BOUND ( 'NONE', #894, .T. ) ;
#14035=ORIENTED_EDGE ( 'NONE', *, *, #14369, .T. ) ;
#14067=DIRECTION ( 'NONE',  ( 0.000000000000000000, 0.000000000000000000, 1.000000000000000000 ) ) ;
#14082=EDGE_LOOP ( 'NONE', ( #5120, #1291 ) ) ;
#14105=ORIENTED_EDGE ( 'NONE', *, *, #15274, .F. ) ;
#14110=VERTEX_POINT ( 'NONE', #3683 ) ;
#14114=CIRCLE ( 'NONE', #9053, 1.999999999999999556 ) ;
#14125=AXIS2_PLACEMENT_3D ( 'NONE', #9475, #798, #12964 ) ;
#14126=DIRECTION ( 'NONE',  ( 0.000000000000000000, 0.000000000000000000, 1.000000000000000000 ) ) ;
#14139=CARTESIAN_POINT ( 'NONE',  ( 1.979652835806277785E-15, -0.001000000000000132727, 11.50000000000000000 ) ) ;
#14141=ORIENTED_EDGE ( 'NONE', *, *, #8685, .F. ) ;
#14154=CARTESIAN_POINT ( 'NONE',  ( 2.449293598294706513E-15, 2.000000000000000000, 20.00000000000000000 ) ) ;
#14180=VERTEX_POINT ( 'NONE', #29 ) ;
#14186=FACE_BOUND ( 'NONE', #1840, .T. ) ;
#14187=VERTEX_POINT ( 'NONE', #3992 ) ;
#14189=EDGE_CURVE ( 'NONE', #9498, #14110, #7337, .T. ) ;
#14199=DIRECTION ( 'NONE',  ( 0.000000000000000000, 1.000000000000000000, 0.000000000000000000 ) ) ;
#14201=AXIS2_PLACEMENT_3D ( 'NONE', #6680, #11513, #1651 ) ;
#14241=EDGE_CURVE ( 'NONE', #8559, #9290, #6170, .T. ) ;
#14265=DIRECTION ( 'NONE',  ( 0.000000000000000000, 1.000000000000000000, 0.000000000000000000 ) ) ;
#14283=EDGE_CURVE ( 'NONE', #6446, #9498, #13852, .T. ) ;
#14307=CIRCLE ( 'NONE', #343, 20.00000000000000000 ) ;
#14322=AXIS2_PLACEMENT_3D ( 'NONE', #7688, #8737, #6436 ) ;
#14347=DIRECTION ( 'NONE',  ( -0.000000000000000000, -1.000000000000000000, -0.000000000000000000 ) ) ;
#14352=EDGE_CURVE ( 'NONE', #12581, #4214, #14956, .T. ) ;
#14361=CIRCLE ( 'NONE', #2688, 1.999999999999999556 ) ;
#14369=EDGE_CURVE ( 'NONE', #12563, #8014, #977, .T. ) ;
#14382=EDGE_CURVE ( 'NONE', #13449, #8559, #5556, .T. ) ;
#14383=CARTESIAN_POINT ( 'NONE',  ( -9.750000000000003553, 22.00000000000000000, -3.401296724241641415E-14 ) ) ;
#14388=EDGE_CURVE ( 'NONE', #5635, #8014, #9102, .T. ) ;
#14398=ORIENTED_EDGE ( 'NONE', *, *, #1654, .T. ) ;
#14424=CIRCLE ( 'NONE', #5303, 20.00000000000000000 ) ;
#14436=AXIS2_PLACEMENT_3D ( 'NONE', #12891, #5439, #644 ) ;
#14442=DIRECTION ( 'NONE',  ( -0.000000000000000000, -1.000000000000000000, -0.000000000000000000 ) ) ;
#14444=( GEOMETRIC_REPRESENTATION_CONTEXT ( 3 ) GLOBAL_UNCERTAINTY_ASSIGNED_CONTEXT ( ( #3448 ) ) GLOBAL_UNIT_ASSIGNED_CONTEXT ( ( #15296, #807, #10364 ) ) REPRESENTATION_CONTEXT ( 'NONE', 'WORKASPACE' ) );
#14466=CARTESIAN_POINT ( 'NONE',  ( 0.000000000000000000, 22.00000000000000000, -5.000000000000000000 ) ) ;
#14469=ORIENTED_EDGE ( 'NONE', *, *, #14382, .T. ) ;
#14492=DIRECTION ( 'NONE',  ( 0.000000000000000000, 0.000000000000000000, 1.000000000000000000 ) ) ;
#14514=LINE ( 'NONE', #4660, #9543 ) ;
#14528=DIRECTION ( 'NONE',  ( 0.000000000000000000, 0.000000000000000000, 1.000000000000000000 ) ) ;
#14551=AXIS2_PLACEMENT_3D ( 'NONE', #5700, #756, #6897 ) ;
#14559=CARTESIAN_POINT ( 'NONE',  ( 1.530808498934191916E-15, 22.00000000000000000, -12.50000000000000355 ) ) ;
#14574=CIRCLE ( 'NONE', #9004, 12.50000000000000355 ) ;
#14598=CARTESIAN_POINT ( 'NONE',  ( 0.000000000000000000, 2.000000000000000000, 0.000000000000000000 ) ) ;
#14661=DIRECTION ( 'NONE',  ( 0.000000000000000000, 0.000000000000000000, 1.000000000000000000 ) ) ;
#14676=AXIS2_PLACEMENT_3D ( 'NONE', #5051, #4898, #4817 ) ;
#14687=ORIENTED_EDGE ( 'NONE', *, *, #9426, .F. ) ;
#14691=CARTESIAN_POINT ( 'NONE',  ( 13.50000000000000000, -0.001000000000000132727, -8.673617379884035472E-16 ) ) ;
#14714=ORIENTED_EDGE ( 'NONE', *, *, #9426, .T. ) ;
#14720=AXIS2_PLACEMENT_3D ( 'NONE', #12815, #3198, #5442 ) ;
#14722=CARTESIAN_POINT ( 'NONE',  ( 0.000000000000000000, 2.000000000000000000, -13.50000000000000000 ) ) ;
#14723=CIRCLE ( 'NONE', #4297, 1.499999999999999556 ) ;
#14750=ORIENTED_EDGE ( 'NONE', *, *, #9440, .F. ) ;
#14754=ADVANCED_FACE ( 'NONE', ( #11605, #9160 ), #11374, .T. ) ;
#14760=DIRECTION ( 'NONE',  ( 0.000000000000000000, 0.000000000000000000, 1.000000000000000000 ) ) ;
#14799=DIRECTION ( 'NONE',  ( -0.000000000000000000, 1.000000000000000000, -0.000000000000000000 ) ) ;
#14824=ORIENTED_EDGE ( 'NONE', *, *, #1717, .F. ) ;
#14875=FACE_OUTER_BOUND ( 'NONE', #4052, .T. ) ;
#14882=EDGE_LOOP ( 'NONE', ( #5998, #5199 ) ) ;
#14903=CARTESIAN_POINT ( 'NONE',  ( -2.897581130414634077E-17, 19.99999999999999645, -9.750000000000003553 ) ) ;
#14923=FACE_OUTER_BOUND ( 'NONE', #8068, .T. ) ;
#14925=CARTESIAN_POINT ( 'NONE',  ( 13.50000000000000000, 2.000000000000000000, -8.673617379884035472E-16 ) ) ;
#14956=CIRCLE ( 'NONE', #14436, 5.000000000000000000 ) ;
#14967=DIRECTION ( 'NONE',  ( 0.000000000000000000, -0.000000000000000000, 1.000000000000000000 ) ) ;
#14971=DIRECTION ( 'NONE',  ( 0.000000000000000000, 0.000000000000000000, 1.000000000000000000 ) ) ;
#15001=ADVANCED_FACE ( 'NONE', ( #10872 ), #9525, .F. ) ;
#15026=FACE_BOUND ( 'NONE', #10635, .T. ) ;
#15029=FILL_AREA_STYLE ('',( #15183 ) ) ;
#15049=DIRECTION ( 'NONE',  ( 0.000000000000000000, 0.000000000000000000, 1.000000000000000000 ) ) ;
#15056=ADVANCED_FACE ( 'NONE', ( #10715 ), #1005, .T. ) ;
#15058=AXIS2_PLACEMENT_3D ( 'NONE', #8699, #13842, #6312 ) ;
#15069=CIRCLE ( 'NONE', #9994, 2.000000000000000000 ) ;
#15100=EDGE_CURVE ( 'NONE', #9290, #3041, #11651, .T. ) ;
#15114=EDGE_LOOP ( 'NONE', ( #8847, #2863 ) ) ;
#15141=FILL_AREA_STYLE_COLOUR ( '', #15223 ) ;
#15144=EDGE_CURVE ( 'NONE', #6851, #2492, #6843, .T. ) ;
#15156=VERTEX_POINT ( 'NONE', #5146 ) ;
#15160=CARTESIAN_POINT ( 'NONE',  ( 0.000000000000000000, 22.00000000000000000, 0.000000000000000000 ) ) ;
#15183=FILL_AREA_STYLE_COLOUR ( '', #4563 ) ;
#15198=ORIENTED_EDGE ( 'NONE', *, *, #5079, .T. ) ;
#15202=AXIS2_PLACEMENT_3D ( 'NONE', #9027, #7972, #4397 ) ;
#15203=LINE ( 'NONE', #9238, #10233 ) ;
#15219=CARTESIAN_POINT ( 'NONE',  ( 2.897581130414634077E-17, 22.00000000000000000, 9.750000000000003553 ) ) ;
#15223=COLOUR_RGB ( '', 0.08235294, 0.09019608, 0.10196078) ;
#15229=ADVANCED_FACE ( 'NONE', ( #2093 ), #2017, .T. ) ;
#15232=ADVANCED_FACE ( 'NONE', ( #14186, #901, #4258, #14033, #5770, #750 ), #1862, .F. ) ;
#15271=CARTESIAN_POINT ( 'NONE',  ( 1.734723475976807094E-15, 0.000000000000000000, 15.50000000000000000 ) ) ;
#15274=EDGE_CURVE ( 'NONE', #1681, #13364, #11404, .T. ) ;
#15276=CARTESIAN_POINT ( 'NONE',  ( -2.897581130414634077E-17, 22.00000000000000000, -9.750000000000003553 ) ) ;
#15296=( LENGTH_UNIT ( ) NAMED_UNIT ( * ) SI_UNIT ( .MILLI., .METRE. ) );
#15300=DIRECTION ( 'NONE',  ( 0.000000000000000000, 0.000000000000000000, 1.000000000000000000 ) ) ;
#15315=PRODUCT_DEFINITION ( 'UNKNOWN', '', #6300, #11500 ) ;
#15337=LINE ( 'NONE', #3083, #6121 ) ;
#15338=ORIENTED_EDGE ( 'NONE', *, *, #275, .T. ) ;
#15340=DIRECTION ( 'NONE',  ( -0.000000000000000000, 1.000000000000000000, -0.000000000000000000 ) ) ;
#15345=LINE ( 'NONE', #13902, #4505 ) ;
#15363=CARTESIAN_POINT ( 'NONE',  ( 2.126728311762493650E-16, 22.00000000000000000, 8.250000000000003553 ) ) ;
#15378=LINE ( 'NONE', #966, #10512 ) ;
#15388=ADVANCED_FACE ( 'NONE', ( #8563 ), #13389, .F. ) ;
#15400=DIRECTION ( 'NONE',  ( 0.000000000000000000, 0.000000000000000000, -1.000000000000000000 ) ) ;
#15417=( LENGTH_UNIT ( ) NAMED_UNIT ( * ) SI_UNIT ( .MILLI., .METRE. ) );
#15422=AXIS2_PLACEMENT_3D ( 'NONE', #3697, #1306, #4985 ) ;
#15426=VERTEX_POINT ( 'NONE', #1608 ) ;
#15441=FACE_OUTER_BOUND ( 'NONE', #7714, .T. ) ;
#15467=ADVANCED_FACE ( 'NONE', ( #2814 ), #13782, .F. ) ;
#15480=EDGE_CURVE ( 'NONE', #3549, #3604, #5322, .T. ) ;
#15484=MANIFOLD_SOLID_BREP ( 'AdvancedHole2', #11562 ) ;
#15494=CIRCLE ( 'NONE', #7817, 20.00000000000000000 ) ;
#15537=DIRECTION ( 'NONE',  ( 0.000000000000000000, 1.000000000000000000, 0.000000000000000000 ) ) ;
#15541=EDGE_CURVE ( 'NONE', #1040, #6081, #5582, .T. ) ;
#15549=ORIENTED_EDGE ( 'NONE', *, *, #15588, .T. ) ;
#15555=EDGE_CURVE ( 'NONE', #9501, #302, #6414, .T. ) ;
#15560=DIRECTION ( 'NONE',  ( 0.000000000000000000, 0.000000000000000000, -1.000000000000000000 ) ) ;
#15575=CARTESIAN_POINT ( 'NONE',  ( 0.000000000000000000, 19.99999999999999645, 0.000000000000000000 ) ) ;
#15588=EDGE_CURVE ( 'NONE', #3604, #3549, #8644, .T. ) ;
#15594=CYLINDRICAL_SURFACE ( 'NONE', #3793, 1.499999999999999556 ) ;
#15609=ORIENTED_EDGE ( 'NONE', *, *, #68, .F. ) ;
#15674=EDGE_CURVE ( 'NONE', #10771, #5182, #15494, .T. ) ;
#15684=ORIENTED_EDGE ( 'NONE', *, *, #11062, .F. ) ;
#15703=DIRECTION ( 'NONE',  ( -0.000000000000000000, -1.000000000000000000, -0.000000000000000000 ) ) ;
#15725=VECTOR ( 'NONE', #4155, 1000.000000000000000 ) ;
ENDSEC;
END-ISO-10303-21;
